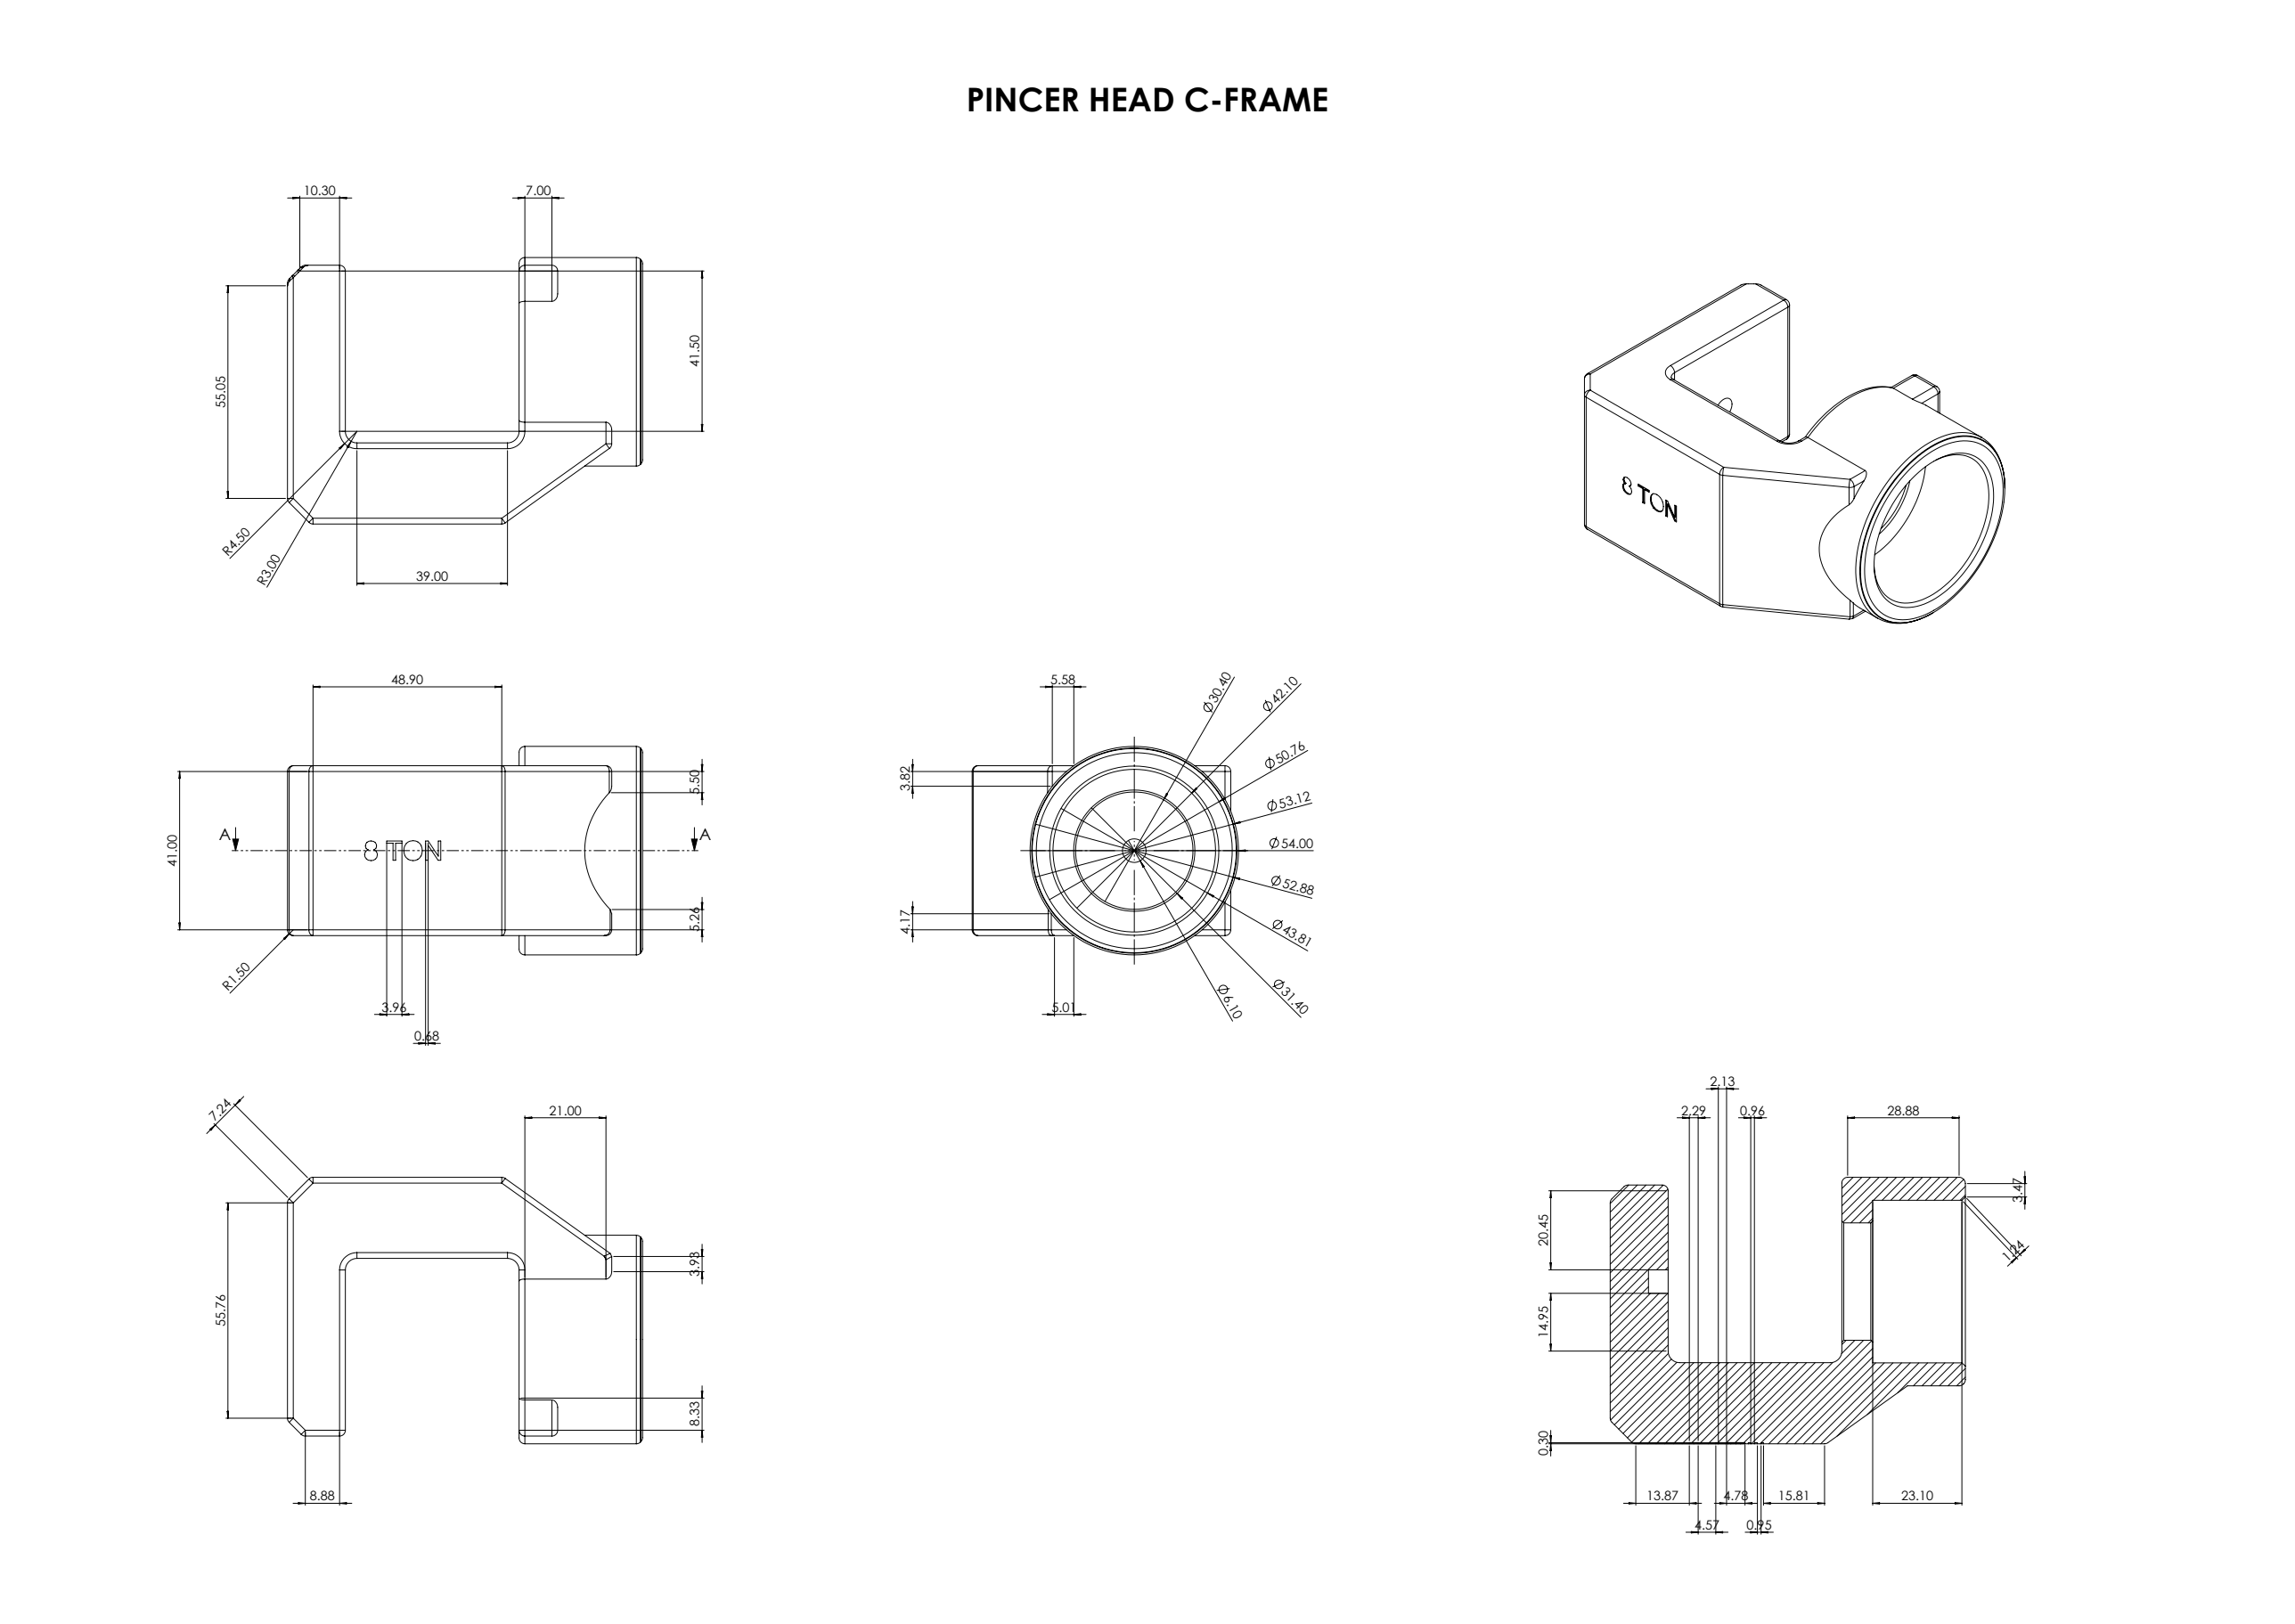
ISO-10303-21;
HEADER;
/* Generated by software containing ST-Developer
 * from STEP Tools, Inc. (www.steptools.com) 
 */

FILE_DESCRIPTION(
/* description */ (''),
/* implementation_level */ '2;1');

FILE_NAME(
/* name */ '01_Pincer_Head_C-Frame.step',
/* time_stamp */ '2026-10-26T03:55:20-07:00',
/* author */ (''),
/* organization */ (''),
/* preprocessor_version */ 'ST-DEVELOPER v20.2',
/* originating_system */ 'Autodesk Translation Framework v15.15.0.0',
/* authorisation */ '');

FILE_SCHEMA (('AUTOMOTIVE_DESIGN { 1 0 10303 214 3 1 1 }'));
ENDSEC;

DATA;
#10=MECHANICAL_DESIGN_GEOMETRIC_PRESENTATION_REPRESENTATION('',(#175),#45236);
#135=SHAPE_REPRESENTATION_RELATIONSHIP('SRR','None',#45314,#155);
#155=ADVANCED_BREP_SHAPE_REPRESENTATION('',(#195),#45216);
#175=STYLED_ITEM('',(#45463),#195);
#195=MANIFOLD_SOLID_BREP('Body1',#16517);
#215=TOROIDAL_SURFACE('',#16890,25.3786796564404,1.5);
#216=TOROIDAL_SURFACE('',#16900,25.5,1.5);
#217=TOROIDAL_SURFACE('',#16910,25.5,1.5);
#218=TOROIDAL_SURFACE('',#16914,4.5,1.5);
#219=TOROIDAL_SURFACE('',#16920,4.5,1.5);
#220=TOROIDAL_SURFACE('',#16924,4.5,1.5);
#221=TOROIDAL_SURFACE('',#16926,25.5,1.5);
#222=TOROIDAL_SURFACE('',#16927,4.5,1.5);
#223=TOROIDAL_SURFACE('',#16932,25.5,1.5);
#231=SPHERICAL_SURFACE('',#16793,1.5);
#232=SPHERICAL_SURFACE('',#16796,1.5);
#233=SPHERICAL_SURFACE('',#16802,1.5);
#234=SPHERICAL_SURFACE('',#16808,1.5);
#235=SPHERICAL_SURFACE('',#16812,1.5);
#236=SPHERICAL_SURFACE('',#16817,1.5);
#237=SPHERICAL_SURFACE('',#16821,1.5);
#238=SPHERICAL_SURFACE('',#16827,1.5);
#239=SPHERICAL_SURFACE('',#16830,1.5);
#240=SPHERICAL_SURFACE('',#16836,1.5);
#241=SPHERICAL_SURFACE('',#16842,1.5);
#242=SPHERICAL_SURFACE('',#16848,1.5);
#243=SPHERICAL_SURFACE('',#16853,1.5);
#244=SPHERICAL_SURFACE('',#16874,1.5);
#245=SPHERICAL_SURFACE('',#16880,1.5);
#246=ELLIPSE('',#16775,30.3654774451956,27.);
#247=ELLIPSE('',#16782,46.4525564420302,27.);
#256=B_SPLINE_CURVE_WITH_KNOTS('',3,(#22232,#22233,#22234,#22235,#22236,
#22237,#22238,#22239,#22240,#22241,#22242,#22243,#22244,#22245,#22246,#22247,
#22248,#22249,#22250,#22251,#22252,#22253,#22254,#22255,#22256,#22257,#22258,
#22259,#22260,#22261,#22262,#22263,#22264,#22265,#22266,#22267,#22268,#22269,
#22270,#22271,#22272,#22273,#22274,#22275,#22276,#22277,#22278,#22279,#22280,
#22281,#22282,#22283,#22284,#22285,#22286),.UNSPECIFIED.,.F.,.F.,(4,3,3,
3,3,3,3,3,3,3,3,3,3,3,3,3,3,3,4),(0.,0.045710607901934,0.0936977578945001,
0.144847111669027,0.20140314890997,0.272909847076527,0.34684212796304,0.403542711042019,
0.454759213428076,0.503663771096975,0.553082777660006,0.60625025134459,
0.667135318470237,0.750351488852678,0.812763616639508,0.865509180697515,
0.91510065731714,0.961342755203381,1.),.UNSPECIFIED.);
#257=B_SPLINE_CURVE_WITH_KNOTS('',3,(#22288,#22289,#22290,#22291),
 .UNSPECIFIED.,.F.,.F.,(4,4),(0.,1.),.UNSPECIFIED.);
#258=B_SPLINE_CURVE_WITH_KNOTS('',3,(#22293,#22294,#22295,#22296,#22297,
#22298,#22299,#22300,#22301,#22302,#22303,#22304,#22305,#22306,#22307,#22308,
#22309,#22310,#22311,#22312,#22313,#22314,#22315,#22316,#22317,#22318,#22319,
#22320,#22321,#22322,#22323,#22324,#22325,#22326,#22327,#22328,#22329,#22330,
#22331,#22332,#22333,#22334,#22335,#22336,#22337,#22338,#22339,#22340,#22341,
#22342,#22343,#22344,#22345,#22346,#22347),.UNSPECIFIED.,.F.,.F.,(4,3,3,
3,3,3,3,3,3,3,3,3,3,3,3,3,3,3,4),(0.,0.0457165824991635,0.0937104844515761,
0.144867913797289,0.201436011576242,0.27297908229306,0.346880659378771,
0.403581201094802,0.454799677982589,0.503723597905468,0.553141531246011,
0.606309913173532,0.667202763475632,0.750402072606724,0.812801554455043,
0.865537008236129,0.915120309500579,0.961355859688362,1.),.UNSPECIFIED.);
#259=B_SPLINE_CURVE_WITH_KNOTS('',3,(#22370,#22371,#22372,#22373,#22374),
 .UNSPECIFIED.,.F.,.F.,(4,1,4),(-1.66265780683826,-0.950090175336147,8.76618254786689E-34),
 .UNSPECIFIED.);
#260=B_SPLINE_CURVE_WITH_KNOTS('',3,(#22377,#22378,#22379,#22380,#22381),
 .UNSPECIFIED.,.F.,.F.,(4,1,4),(-8.76618254786689E-34,0.950090175336147,
1.66265780683826),.UNSPECIFIED.);
#261=B_SPLINE_CURVE_WITH_KNOTS('',3,(#22452,#22453,#22454,#22455,#22456,
#22457,#22458,#22459,#22460,#22461,#22462,#22463,#22464,#22465,#22466,#22467,
#22468,#22469,#22470,#22471,#22472,#22473,#22474,#22475,#22476,#22477,#22478,
#22479,#22480,#22481,#22482,#22483,#22484,#22485,#22486,#22487,#22488,#22489,
#22490,#22491,#22492,#22493,#22494,#22495,#22496,#22497,#22498,#22499,#22500,
#22501,#22502,#22503,#22504,#22505,#22506),.UNSPECIFIED.,.F.,.F.,(4,3,3,
3,3,3,3,3,3,3,3,3,3,3,3,3,3,3,4),(0.,0.0454739962515773,0.0931998981823239,
0.144047233375039,0.200179420009566,0.270609269371814,0.345305256937859,
0.401904934183246,0.452978957125852,0.503375918080837,0.552516920031195,
0.605334615481369,0.665679077650195,0.749259308237646,0.811944481178235,
0.864470546131162,0.91385478632005,0.959883517726927,1.),.UNSPECIFIED.);
#262=B_SPLINE_CURVE_WITH_KNOTS('',3,(#22508,#22509,#22510,#22511),
 .UNSPECIFIED.,.F.,.F.,(4,4),(-1.,0.),.UNSPECIFIED.);
#263=B_SPLINE_CURVE_WITH_KNOTS('',3,(#22513,#22514,#22515,#22516,#22517,
#22518,#22519,#22520,#22521,#22522,#22523,#22524,#22525,#22526,#22527,#22528,
#22529,#22530,#22531,#22532,#22533,#22534,#22535,#22536,#22537,#22538,#22539,
#22540,#22541,#22542,#22543,#22544,#22545,#22546,#22547,#22548,#22549,#22550,
#22551,#22552,#22553,#22554,#22555,#22556,#22557,#22558,#22559,#22560,#22561,
#22562,#22563,#22564,#22565,#22566,#22567),.UNSPECIFIED.,.F.,.F.,(4,3,3,
3,3,3,3,3,3,3,3,3,3,3,3,3,3,3,4),(0.,0.0454759500687694,0.0932040608878028,
0.144054037760376,0.200190152021456,0.270631477875933,0.345316813881959,
0.401916574351127,0.452991295574466,0.503400827180246,0.552541816304096,
0.605360167195349,0.665708324703348,0.749281243527511,0.811960932645634,
0.864483394812729,0.913864760430574,0.959891262991555,1.),.UNSPECIFIED.);
#264=B_SPLINE_CURVE_WITH_KNOTS('',3,(#22595,#22596,#22597,#22598,#22599,
#22600,#22601,#22602,#22603,#22604,#22605,#22606,#22607,#22608,#22609,#22610,
#22611,#22612,#22613,#22614,#22615,#22616,#22617,#22618,#22619,#22620,#22621,
#22622,#22623,#22624,#22625,#22626,#22627,#22628,#22629,#22630,#22631,#22632,
#22633,#22634,#22635,#22636,#22637,#22638,#22639,#22640,#22641,#22642,#22643,
#22644,#22645,#22646,#22647,#22648,#22649),.UNSPECIFIED.,.F.,.F.,(4,3,3,
3,3,3,3,3,3,3,3,3,3,3,3,3,3,3,4),(0.,0.0454739962517236,0.0931998981821424,
0.144047233377289,0.200179420014148,0.270609269376805,0.345305256939856,
0.401904934184723,0.452978957126951,0.503375918082738,0.552516920034218,
0.605334615484988,0.665679077654914,0.749259308241186,0.811944481180889,
0.864470546134333,0.913854786323009,0.959883517729389,1.),.UNSPECIFIED.);
#265=B_SPLINE_CURVE_WITH_KNOTS('',3,(#22651,#22652,#22653,#22654),
 .UNSPECIFIED.,.F.,.F.,(4,4),(0.,1.),.UNSPECIFIED.);
#266=B_SPLINE_CURVE_WITH_KNOTS('',3,(#22656,#22657,#22658,#22659,#22660,
#22661,#22662,#22663,#22664,#22665,#22666,#22667,#22668,#22669,#22670,#22671,
#22672,#22673,#22674,#22675,#22676,#22677,#22678,#22679,#22680,#22681,#22682,
#22683,#22684,#22685,#22686,#22687,#22688,#22689,#22690,#22691,#22692,#22693,
#22694,#22695,#22696,#22697,#22698,#22699,#22700,#22701,#22702,#22703,#22704,
#22705,#22706,#22707,#22708,#22709,#22710),.UNSPECIFIED.,.F.,.F.,(4,3,3,
3,3,3,3,3,3,3,3,3,3,3,3,3,3,3,4),(0.,0.0454759500669044,0.0932040608838389,
0.144054037755869,0.200190152008621,0.270631477848411,0.345316813870146,
0.401916574343999,0.4529912955674,0.503400827166756,0.552541816289859,0.605360167180691,
0.665708324686459,0.749281243514844,0.811960932636133,0.864483394804765,
0.913864760422638,0.959891262983851,1.),.UNSPECIFIED.);
#267=B_SPLINE_CURVE_WITH_KNOTS('',3,(#22729,#22730,#22731,#22732),
 .UNSPECIFIED.,.F.,.F.,(4,4),(1.38548660592135,2.14032342811115),
 .UNSPECIFIED.);
#268=B_SPLINE_CURVE_WITH_KNOTS('',3,(#22735,#22736,#22737,#22738),
 .UNSPECIFIED.,.F.,.F.,(4,4),(-2.14032342811115,-1.38548660592135),
 .UNSPECIFIED.);
#269=B_SPLINE_CURVE_WITH_KNOTS('',3,(#22759,#22760,#22761,#22762),
 .UNSPECIFIED.,.F.,.F.,(4,4),(-1.33701776267244,-0.785398163397445),
 .UNSPECIFIED.);
#270=B_SPLINE_CURVE_WITH_KNOTS('',3,(#22765,#22766,#22767,#22768),
 .UNSPECIFIED.,.F.,.F.,(4,4),(0.785398163397445,1.33701776267244),
 .UNSPECIFIED.);
#271=B_SPLINE_CURVE_WITH_KNOTS('',3,(#22785,#22786,#22787,#22788),
 .UNSPECIFIED.,.F.,.F.,(4,4),(-2.35619449019235,-2.14032342811107),
 .UNSPECIFIED.);
#272=B_SPLINE_CURVE_WITH_KNOTS('',3,(#22789,#22790,#22791,#22792),
 .UNSPECIFIED.,.F.,.F.,(4,4),(2.14032342811107,2.35619449019235),
 .UNSPECIFIED.);
#273=B_SPLINE_CURVE_WITH_KNOTS('',3,(#22818,#22819,#22820,#22821),
 .UNSPECIFIED.,.F.,.F.,(4,4),(-1.5707963267949,-1.33701776267243),
 .UNSPECIFIED.);
#274=B_SPLINE_CURVE_WITH_KNOTS('',3,(#22822,#22823,#22824,#22825),
 .UNSPECIFIED.,.F.,.F.,(4,4),(1.33701776267243,1.5707963267949),
 .UNSPECIFIED.);
#275=B_SPLINE_CURVE_WITH_KNOTS('',3,(#22846,#22847,#22848,#22849),
 .UNSPECIFIED.,.F.,.F.,(4,4),(-1.33701776267244,-0.785398163397449),
 .UNSPECIFIED.);
#276=B_SPLINE_CURVE_WITH_KNOTS('',3,(#22852,#22853,#22854,#22855),
 .UNSPECIFIED.,.F.,.F.,(4,4),(0.785398163397449,1.33701776267244),
 .UNSPECIFIED.);
#277=B_SPLINE_CURVE_WITH_KNOTS('',3,(#22872,#22873,#22874,#22875),
 .UNSPECIFIED.,.F.,.F.,(4,4),(1.33701776267244,1.5707963267949),
 .UNSPECIFIED.);
#278=B_SPLINE_CURVE_WITH_KNOTS('',3,(#22876,#22877,#22878,#22879),
 .UNSPECIFIED.,.F.,.F.,(4,4),(-1.5707963267949,-1.33701776267244),
 .UNSPECIFIED.);
#279=B_SPLINE_CURVE_WITH_KNOTS('',3,(#22897,#22898,#22899,#22900),
 .UNSPECIFIED.,.F.,.F.,(4,4),(1.38548660592135,2.14032342811115),
 .UNSPECIFIED.);
#280=B_SPLINE_CURVE_WITH_KNOTS('',3,(#22903,#22904,#22905,#22906),
 .UNSPECIFIED.,.F.,.F.,(4,4),(-2.14032342811115,-1.38548660592135),
 .UNSPECIFIED.);
#281=B_SPLINE_CURVE_WITH_KNOTS('',3,(#22923,#22924,#22925,#22926),
 .UNSPECIFIED.,.F.,.F.,(4,4),(2.14032342811108,2.35619449019234),
 .UNSPECIFIED.);
#282=B_SPLINE_CURVE_WITH_KNOTS('',3,(#22927,#22928,#22929,#22930),
 .UNSPECIFIED.,.F.,.F.,(4,4),(-2.35619449019234,-2.14032342811108),
 .UNSPECIFIED.);
#283=B_SPLINE_CURVE_WITH_KNOTS('',3,(#22971,#22972,#22973,#22974,#22975,
#22976,#22977,#22978,#22979,#22980,#22981,#22982),.UNSPECIFIED.,.F.,.F.,
(4,2,2,2,2,4),(0.,0.0283853554165653,0.0567707108331306,0.113541421666261,
0.206773466476135,0.300005511286008),.UNSPECIFIED.);
#284=B_SPLINE_CURVE_WITH_KNOTS('',3,(#22988,#22989,#22990,#22991,#22992,
#22993,#22994,#22995,#22996,#22997),.UNSPECIFIED.,.F.,.F.,(4,2,2,2,4),(0.328734721229726,
0.593926356430402,0.667111024695369,0.687829707063932,0.708548389432494),
 .UNSPECIFIED.);
#285=B_SPLINE_CURVE_WITH_KNOTS('',3,(#23011,#23012,#23013,#23014,#23015,
#23016,#23017,#23018),.UNSPECIFIED.,.F.,.F.,(4,2,2,4),(0.894852523096926,
0.994118550241906,1.09338457738688,1.10550146254272),.UNSPECIFIED.);
#286=B_SPLINE_CURVE_WITH_KNOTS('',3,(#23023,#23024,#23025,#23026,#23027,
#23028,#23029,#23030,#23031,#23032,#23033,#23034),.UNSPECIFIED.,.F.,.F.,
(4,2,2,2,2,4),(0.,0.0283853554165652,0.0567707108331305,0.113541421666261,
0.206773466476134,0.300005511286007),.UNSPECIFIED.);
#287=B_SPLINE_CURVE_WITH_KNOTS('',2,(#23117,#23118,#23119),
 .UNSPECIFIED.,.F.,.F.,(3,3),(0.,1.),.UNSPECIFIED.);
#288=B_SPLINE_CURVE_WITH_KNOTS('',2,(#23121,#23122,#23123),
 .UNSPECIFIED.,.F.,.F.,(3,3),(0.,1.),.UNSPECIFIED.);
#289=B_SPLINE_CURVE_WITH_KNOTS('',2,(#23125,#23126,#23127),
 .UNSPECIFIED.,.F.,.F.,(3,3),(0.,1.),.UNSPECIFIED.);
#290=B_SPLINE_CURVE_WITH_KNOTS('',2,(#23129,#23130,#23131),
 .UNSPECIFIED.,.F.,.F.,(3,3),(0.,1.),.UNSPECIFIED.);
#291=B_SPLINE_CURVE_WITH_KNOTS('',2,(#23133,#23134,#23135),
 .UNSPECIFIED.,.F.,.F.,(3,3),(0.,1.),.UNSPECIFIED.);
#292=B_SPLINE_CURVE_WITH_KNOTS('',2,(#23137,#23138,#23139),
 .UNSPECIFIED.,.F.,.F.,(3,3),(0.,1.),.UNSPECIFIED.);
#293=B_SPLINE_CURVE_WITH_KNOTS('',2,(#23141,#23142,#23143),
 .UNSPECIFIED.,.F.,.F.,(3,3),(0.,1.),.UNSPECIFIED.);
#294=B_SPLINE_CURVE_WITH_KNOTS('',2,(#23145,#23146,#23147),
 .UNSPECIFIED.,.F.,.F.,(3,3),(0.,1.),.UNSPECIFIED.);
#295=B_SPLINE_CURVE_WITH_KNOTS('',2,(#23149,#23150,#23151),
 .UNSPECIFIED.,.F.,.F.,(3,3),(0.,1.),.UNSPECIFIED.);
#296=B_SPLINE_CURVE_WITH_KNOTS('',2,(#23153,#23154,#23155),
 .UNSPECIFIED.,.F.,.F.,(3,3),(0.,1.),.UNSPECIFIED.);
#297=B_SPLINE_CURVE_WITH_KNOTS('',2,(#23156,#23157,#23158),
 .UNSPECIFIED.,.F.,.F.,(3,3),(0.,1.),.UNSPECIFIED.);
#298=B_SPLINE_CURVE_WITH_KNOTS('',2,(#23177,#23178,#23179),
 .UNSPECIFIED.,.F.,.F.,(3,3),(0.,1.),.UNSPECIFIED.);
#299=B_SPLINE_CURVE_WITH_KNOTS('',2,(#23181,#23182,#23183),
 .UNSPECIFIED.,.F.,.F.,(3,3),(0.,1.),.UNSPECIFIED.);
#300=B_SPLINE_CURVE_WITH_KNOTS('',2,(#23185,#23186,#23187),
 .UNSPECIFIED.,.F.,.F.,(3,3),(0.,1.),.UNSPECIFIED.);
#301=B_SPLINE_CURVE_WITH_KNOTS('',2,(#23189,#23190,#23191),
 .UNSPECIFIED.,.F.,.F.,(3,3),(0.,1.),.UNSPECIFIED.);
#302=B_SPLINE_CURVE_WITH_KNOTS('',2,(#23193,#23194,#23195),
 .UNSPECIFIED.,.F.,.F.,(3,3),(0.,1.),.UNSPECIFIED.);
#303=B_SPLINE_CURVE_WITH_KNOTS('',2,(#23197,#23198,#23199),
 .UNSPECIFIED.,.F.,.F.,(3,3),(0.,1.),.UNSPECIFIED.);
#304=B_SPLINE_CURVE_WITH_KNOTS('',2,(#23201,#23202,#23203),
 .UNSPECIFIED.,.F.,.F.,(3,3),(0.,1.),.UNSPECIFIED.);
#305=B_SPLINE_CURVE_WITH_KNOTS('',2,(#23205,#23206,#23207),
 .UNSPECIFIED.,.F.,.F.,(3,3),(0.,1.),.UNSPECIFIED.);
#306=B_SPLINE_CURVE_WITH_KNOTS('',2,(#23209,#23210,#23211),
 .UNSPECIFIED.,.F.,.F.,(3,3),(0.,1.),.UNSPECIFIED.);
#307=B_SPLINE_CURVE_WITH_KNOTS('',2,(#23213,#23214,#23215),
 .UNSPECIFIED.,.F.,.F.,(3,3),(0.,1.),.UNSPECIFIED.);
#308=B_SPLINE_CURVE_WITH_KNOTS('',2,(#23217,#23218,#23219),
 .UNSPECIFIED.,.F.,.F.,(3,3),(0.,1.),.UNSPECIFIED.);
#309=B_SPLINE_CURVE_WITH_KNOTS('',2,(#23221,#23222,#23223),
 .UNSPECIFIED.,.F.,.F.,(3,3),(0.,1.),.UNSPECIFIED.);
#310=B_SPLINE_CURVE_WITH_KNOTS('',2,(#23225,#23226,#23227),
 .UNSPECIFIED.,.F.,.F.,(3,3),(0.,1.),.UNSPECIFIED.);
#311=B_SPLINE_CURVE_WITH_KNOTS('',2,(#23229,#23230,#23231),
 .UNSPECIFIED.,.F.,.F.,(3,3),(0.,1.),.UNSPECIFIED.);
#312=B_SPLINE_CURVE_WITH_KNOTS('',2,(#23233,#23234,#23235),
 .UNSPECIFIED.,.F.,.F.,(3,3),(0.,1.),.UNSPECIFIED.);
#313=B_SPLINE_CURVE_WITH_KNOTS('',2,(#23236,#23237,#23238),
 .UNSPECIFIED.,.F.,.F.,(3,3),(0.,1.),.UNSPECIFIED.);
#314=B_SPLINE_CURVE_WITH_KNOTS('',3,(#23280,#23281,#23282,#23283,#23284,
#23285,#23286,#23287,#23288,#23289,#23290,#23291),.UNSPECIFIED.,.F.,.F.,
(4,2,2,2,2,4),(-0.300005511286007,-0.206773466476134,-0.113541421666261,
-0.0567707108331306,-0.0283853554165654,0.),.UNSPECIFIED.);
#315=B_SPLINE_CURVE_WITH_KNOTS('',3,(#23300,#23301,#23302,#23303,#23304,
#23305,#23306,#23307,#23308,#23309,#23310,#23311,#23312,#23313),
 .UNSPECIFIED.,.F.,.F.,(4,2,2,2,2,2,4),(-0.242126305586689,-0.241475938992465,
-0.207325141862153,-0.17328250313445,-0.113202201999937,-0.0559588482258517,
0.),.UNSPECIFIED.);
#316=B_SPLINE_CURVE_WITH_KNOTS('',3,(#23315,#23316,#23317,#23318,#23319,
#23320,#23321,#23322,#23323,#23324,#23325,#23326,#23327,#23328),
 .UNSPECIFIED.,.F.,.F.,(4,2,2,2,2,2,4),(-0.237971793841113,-0.180365854109777,
-0.122215701674832,-0.0629296381239613,-0.0314884565302302,0.,0.000668991455295416),
 .UNSPECIFIED.);
#317=B_SPLINE_CURVE_WITH_KNOTS('',3,(#23339,#23340,#23341,#23342,#23343,
#23344,#23345,#23346,#23347,#23348,#23349,#23350,#23351,#23352),
 .UNSPECIFIED.,.F.,.F.,(4,2,2,2,2,2,4),(-0.23846990825455,-0.237798685175548,
-0.20633335283318,-0.174914932942728,-0.115672316276476,-0.0575645322663487,
0.),.UNSPECIFIED.);
#318=B_SPLINE_CURVE_WITH_KNOTS('',3,(#23356,#23357,#23358,#23359,#23360,
#23361,#23362,#23363,#23364,#23365,#23366,#23367,#23368,#23369),
 .UNSPECIFIED.,.F.,.F.,(4,2,2,2,2,2,4),(-0.241896356494029,-0.185842740394847,
-0.128518974500819,-0.0683631385924297,-0.0342301099048936,0.,0.000659700792702867),
 .UNSPECIFIED.);
#319=B_SPLINE_CURVE_WITH_KNOTS('',3,(#23388,#23389,#23390,#23391,#23392,
#23393,#23394,#23395,#23396,#23397),.UNSPECIFIED.,.F.,.F.,(4,2,2,2,4),(0.712943458944601,
0.733662141313163,0.754380823681726,0.827565491946693,1.09275712714737),
 .UNSPECIFIED.);
#320=B_SPLINE_CURVE_WITH_KNOTS('',3,(#23402,#23403,#23404,#23405,#23406,
#23407,#23408,#23409,#23410,#23411,#23412,#23413),.UNSPECIFIED.,.F.,.F.,
(4,2,2,2,2,4),(-0.300005511286008,-0.206773466476135,-0.113541421666261,
-0.0567707108331308,-0.0283853554165654,0.),.UNSPECIFIED.);
#321=B_SPLINE_CURVE_WITH_KNOTS('',3,(#23474,#23475,#23476,#23477,#23478,
#23479,#23480,#23481,#23482,#23483,#23484,#23485,#23486,#23487),
 .UNSPECIFIED.,.F.,.F.,(4,2,2,2,2,2,4),(-0.000578412997427686,0.,0.0341328715078763,
0.0680999028359124,0.128446519154858,0.185899361060066,0.241981137339067),
 .UNSPECIFIED.);
#322=B_SPLINE_CURVE_WITH_KNOTS('',3,(#23498,#23499,#23500,#23501,#23502,
#23503,#23504,#23505,#23506,#23507,#23508,#23509,#23510,#23511),
 .UNSPECIFIED.,.F.,.F.,(4,2,2,2,2,2,4),(0.,0.0559818727072018,0.113332368636633,
0.173571484036089,0.207478006800184,0.241550074317809,0.242127456935271),
 .UNSPECIFIED.);
#323=B_SPLINE_CURVE_WITH_KNOTS('',2,(#23531,#23532,#23533),
 .UNSPECIFIED.,.F.,.F.,(3,3),(0.,1.),.UNSPECIFIED.);
#324=B_SPLINE_CURVE_WITH_KNOTS('',2,(#23543,#23544,#23545),
 .UNSPECIFIED.,.F.,.F.,(3,3),(0.,1.),.UNSPECIFIED.);
#325=B_SPLINE_CURVE_WITH_KNOTS('',2,(#23554,#23555,#23556),
 .UNSPECIFIED.,.F.,.F.,(3,3),(0.,1.),.UNSPECIFIED.);
#326=B_SPLINE_CURVE_WITH_KNOTS('',2,(#23565,#23566,#23567),
 .UNSPECIFIED.,.F.,.F.,(3,3),(0.,1.),.UNSPECIFIED.);
#327=B_SPLINE_CURVE_WITH_KNOTS('',2,(#23576,#23577,#23578),
 .UNSPECIFIED.,.F.,.F.,(3,3),(0.,1.),.UNSPECIFIED.);
#328=B_SPLINE_CURVE_WITH_KNOTS('',2,(#23587,#23588,#23589),
 .UNSPECIFIED.,.F.,.F.,(3,3),(0.,1.),.UNSPECIFIED.);
#329=B_SPLINE_CURVE_WITH_KNOTS('',2,(#23598,#23599,#23600),
 .UNSPECIFIED.,.F.,.F.,(3,3),(0.,1.),.UNSPECIFIED.);
#330=B_SPLINE_CURVE_WITH_KNOTS('',2,(#23609,#23610,#23611),
 .UNSPECIFIED.,.F.,.F.,(3,3),(0.,1.),.UNSPECIFIED.);
#331=B_SPLINE_CURVE_WITH_KNOTS('',2,(#23620,#23621,#23622),
 .UNSPECIFIED.,.F.,.F.,(3,3),(0.,1.),.UNSPECIFIED.);
#332=B_SPLINE_CURVE_WITH_KNOTS('',2,(#23631,#23632,#23633),
 .UNSPECIFIED.,.F.,.F.,(3,3),(0.,1.),.UNSPECIFIED.);
#333=B_SPLINE_CURVE_WITH_KNOTS('',2,(#23640,#23641,#23642),
 .UNSPECIFIED.,.F.,.F.,(3,3),(0.,1.),.UNSPECIFIED.);
#334=B_SPLINE_CURVE_WITH_KNOTS('',2,(#23686,#23687,#23688),
 .UNSPECIFIED.,.F.,.F.,(3,3),(0.,1.),.UNSPECIFIED.);
#335=B_SPLINE_CURVE_WITH_KNOTS('',2,(#23698,#23699,#23700),
 .UNSPECIFIED.,.F.,.F.,(3,3),(0.,1.),.UNSPECIFIED.);
#336=B_SPLINE_CURVE_WITH_KNOTS('',2,(#23709,#23710,#23711),
 .UNSPECIFIED.,.F.,.F.,(3,3),(0.,1.),.UNSPECIFIED.);
#337=B_SPLINE_CURVE_WITH_KNOTS('',2,(#23720,#23721,#23722),
 .UNSPECIFIED.,.F.,.F.,(3,3),(0.,1.),.UNSPECIFIED.);
#338=B_SPLINE_CURVE_WITH_KNOTS('',2,(#23731,#23732,#23733),
 .UNSPECIFIED.,.F.,.F.,(3,3),(0.,1.),.UNSPECIFIED.);
#339=B_SPLINE_CURVE_WITH_KNOTS('',2,(#23742,#23743,#23744),
 .UNSPECIFIED.,.F.,.F.,(3,3),(0.,1.),.UNSPECIFIED.);
#340=B_SPLINE_CURVE_WITH_KNOTS('',2,(#23753,#23754,#23755),
 .UNSPECIFIED.,.F.,.F.,(3,3),(0.,1.),.UNSPECIFIED.);
#341=B_SPLINE_CURVE_WITH_KNOTS('',2,(#23764,#23765,#23766),
 .UNSPECIFIED.,.F.,.F.,(3,3),(0.,1.),.UNSPECIFIED.);
#342=B_SPLINE_CURVE_WITH_KNOTS('',2,(#23775,#23776,#23777),
 .UNSPECIFIED.,.F.,.F.,(3,3),(0.,1.),.UNSPECIFIED.);
#343=B_SPLINE_CURVE_WITH_KNOTS('',2,(#23786,#23787,#23788),
 .UNSPECIFIED.,.F.,.F.,(3,3),(0.,1.),.UNSPECIFIED.);
#344=B_SPLINE_CURVE_WITH_KNOTS('',2,(#23797,#23798,#23799),
 .UNSPECIFIED.,.F.,.F.,(3,3),(0.,1.),.UNSPECIFIED.);
#345=B_SPLINE_CURVE_WITH_KNOTS('',2,(#23808,#23809,#23810),
 .UNSPECIFIED.,.F.,.F.,(3,3),(0.,1.),.UNSPECIFIED.);
#346=B_SPLINE_CURVE_WITH_KNOTS('',2,(#23819,#23820,#23821),
 .UNSPECIFIED.,.F.,.F.,(3,3),(0.,1.),.UNSPECIFIED.);
#347=B_SPLINE_CURVE_WITH_KNOTS('',2,(#23830,#23831,#23832),
 .UNSPECIFIED.,.F.,.F.,(3,3),(0.,1.),.UNSPECIFIED.);
#348=B_SPLINE_CURVE_WITH_KNOTS('',2,(#23841,#23842,#23843),
 .UNSPECIFIED.,.F.,.F.,(3,3),(0.,1.),.UNSPECIFIED.);
#349=B_SPLINE_CURVE_WITH_KNOTS('',2,(#23850,#23851,#23852),
 .UNSPECIFIED.,.F.,.F.,(3,3),(0.,1.),.UNSPECIFIED.);
#814=B_SPLINE_SURFACE_WITH_KNOTS('',3,3,((#22206,#22207,#22208,#22209,#22210,
#22211),(#22212,#22213,#22214,#22215,#22216,#22217),(#22218,#22219,#22220,
#22221,#22222,#22223),(#22224,#22225,#22226,#22227,#22228,#22229)),
 .UNSPECIFIED.,.F.,.F.,.F.,(4,4),(4,1,1,4),(0.,1.),(0.,0.571428571428571,
0.857142857142857,1.),.UNSPECIFIED.);
#815=B_SPLINE_SURFACE_WITH_KNOTS('',3,3,((#22349,#22350,#22351,#22352,#22353),
(#22354,#22355,#22356,#22357,#22358),(#22359,#22360,#22361,#22362,#22363),
(#22364,#22365,#22366,#22367,#22368)),.UNSPECIFIED.,.F.,.F.,.F.,(4,4),(4,
1,4),(0.,1.),(-1.66265780683826,-0.950090175336147,8.76618254786689E-34),
 .UNSPECIFIED.);
#816=B_SPLINE_SURFACE_WITH_KNOTS('',3,3,((#22426,#22427,#22428,#22429,#22430,
#22431),(#22432,#22433,#22434,#22435,#22436,#22437),(#22438,#22439,#22440,
#22441,#22442,#22443),(#22444,#22445,#22446,#22447,#22448,#22449)),
 .UNSPECIFIED.,.F.,.F.,.F.,(4,4),(4,1,1,4),(0.,1.),(0.,0.571428571428571,
0.857142857142857,1.),.UNSPECIFIED.);
#817=B_SPLINE_SURFACE_WITH_KNOTS('',3,3,((#22569,#22570,#22571,#22572,#22573,
#22574),(#22575,#22576,#22577,#22578,#22579,#22580),(#22581,#22582,#22583,
#22584,#22585,#22586),(#22587,#22588,#22589,#22590,#22591,#22592)),
 .UNSPECIFIED.,.F.,.F.,.F.,(4,4),(4,1,1,4),(0.,1.),(0.,0.571428571428571,
0.857142857142857,1.),.UNSPECIFIED.);
#818=B_SPLINE_SURFACE_WITH_KNOTS('',3,3,((#22712,#22713,#22714,#22715),
(#22716,#22717,#22718,#22719),(#22720,#22721,#22722,#22723),(#22724,#22725,
#22726,#22727)),.UNSPECIFIED.,.F.,.F.,.F.,(4,4),(4,4),(0.,1.),(1.38548660592135,
2.14032342811115),.UNSPECIFIED.);
#819=B_SPLINE_SURFACE_WITH_KNOTS('',3,3,((#22739,#22740,#22741,#22742),
(#22743,#22744,#22745,#22746),(#22747,#22748,#22749,#22750),(#22751,#22752,
#22753,#22754)),.UNSPECIFIED.,.F.,.F.,.F.,(4,4),(4,4),(0.,1.),(-1.33701776267244,
-0.785398163397445),.UNSPECIFIED.);
#820=B_SPLINE_SURFACE_WITH_KNOTS('',3,3,((#22769,#22770,#22771,#22772),
(#22773,#22774,#22775,#22776),(#22777,#22778,#22779,#22780),(#22781,#22782,
#22783,#22784)),.UNSPECIFIED.,.F.,.F.,.F.,(4,4),(4,4),(0.,1.),(2.14032342811107,
2.35619449019235),.UNSPECIFIED.);
#821=B_SPLINE_SURFACE_WITH_KNOTS('',3,3,((#22802,#22803,#22804,#22805),
(#22806,#22807,#22808,#22809),(#22810,#22811,#22812,#22813),(#22814,#22815,
#22816,#22817)),.UNSPECIFIED.,.F.,.F.,.F.,(4,4),(4,4),(0.,1.),(1.33701776267243,
1.5707963267949),.UNSPECIFIED.);
#822=B_SPLINE_SURFACE_WITH_KNOTS('',3,3,((#22826,#22827,#22828,#22829),
(#22830,#22831,#22832,#22833),(#22834,#22835,#22836,#22837),(#22838,#22839,
#22840,#22841)),.UNSPECIFIED.,.F.,.F.,.F.,(4,4),(4,4),(0.,1.),(0.785398163397449,
1.33701776267244),.UNSPECIFIED.);
#823=B_SPLINE_SURFACE_WITH_KNOTS('',3,3,((#22856,#22857,#22858,#22859),
(#22860,#22861,#22862,#22863),(#22864,#22865,#22866,#22867),(#22868,#22869,
#22870,#22871)),.UNSPECIFIED.,.F.,.F.,.F.,(4,4),(4,4),(0.,1.),(-1.5707963267949,
-1.33701776267244),.UNSPECIFIED.);
#824=B_SPLINE_SURFACE_WITH_KNOTS('',3,3,((#22880,#22881,#22882,#22883),
(#22884,#22885,#22886,#22887),(#22888,#22889,#22890,#22891),(#22892,#22893,
#22894,#22895)),.UNSPECIFIED.,.F.,.F.,.F.,(4,4),(4,4),(0.,1.),(-2.14032342811115,
-1.38548660592135),.UNSPECIFIED.);
#825=B_SPLINE_SURFACE_WITH_KNOTS('',3,3,((#22907,#22908,#22909,#22910),
(#22911,#22912,#22913,#22914),(#22915,#22916,#22917,#22918),(#22919,#22920,
#22921,#22922)),.UNSPECIFIED.,.F.,.F.,.F.,(4,4),(4,4),(0.,1.),(-2.35619449019234,
-2.14032342811108),.UNSPECIFIED.);
#826=B_SPLINE_SURFACE_WITH_KNOTS('',2,1,((#23522,#23523),(#23524,#23525),
(#23526,#23527)),.UNSPECIFIED.,.F.,.F.,.F.,(3,3),(2,2),(0.,1.),(0.,0.0300000000000002),
 .UNSPECIFIED.);
#827=B_SPLINE_SURFACE_WITH_KNOTS('',2,1,((#23535,#23536),(#23537,#23538),
(#23539,#23540)),.UNSPECIFIED.,.F.,.F.,.F.,(3,3),(2,2),(0.,1.),(0.,0.0300000000000002),
 .UNSPECIFIED.);
#828=B_SPLINE_SURFACE_WITH_KNOTS('',2,1,((#23546,#23547),(#23548,#23549),
(#23550,#23551)),.UNSPECIFIED.,.F.,.F.,.F.,(3,3),(2,2),(0.,1.),(0.,0.0300000000000002),
 .UNSPECIFIED.);
#829=B_SPLINE_SURFACE_WITH_KNOTS('',2,1,((#23557,#23558),(#23559,#23560),
(#23561,#23562)),.UNSPECIFIED.,.F.,.F.,.F.,(3,3),(2,2),(0.,1.),(0.,0.0300000000000002),
 .UNSPECIFIED.);
#830=B_SPLINE_SURFACE_WITH_KNOTS('',2,1,((#23568,#23569),(#23570,#23571),
(#23572,#23573)),.UNSPECIFIED.,.F.,.F.,.F.,(3,3),(2,2),(0.,1.),(0.,0.0300000000000002),
 .UNSPECIFIED.);
#831=B_SPLINE_SURFACE_WITH_KNOTS('',2,1,((#23579,#23580),(#23581,#23582),
(#23583,#23584)),.UNSPECIFIED.,.F.,.F.,.F.,(3,3),(2,2),(0.,1.),(0.,0.0300000000000002),
 .UNSPECIFIED.);
#832=B_SPLINE_SURFACE_WITH_KNOTS('',2,1,((#23590,#23591),(#23592,#23593),
(#23594,#23595)),.UNSPECIFIED.,.F.,.F.,.F.,(3,3),(2,2),(0.,1.),(0.,0.0300000000000002),
 .UNSPECIFIED.);
#833=B_SPLINE_SURFACE_WITH_KNOTS('',2,1,((#23601,#23602),(#23603,#23604),
(#23605,#23606)),.UNSPECIFIED.,.F.,.F.,.F.,(3,3),(2,2),(0.,1.),(0.,0.0300000000000002),
 .UNSPECIFIED.);
#834=B_SPLINE_SURFACE_WITH_KNOTS('',2,1,((#23612,#23613),(#23614,#23615),
(#23616,#23617)),.UNSPECIFIED.,.F.,.F.,.F.,(3,3),(2,2),(0.,1.),(0.,0.0300000000000002),
 .UNSPECIFIED.);
#835=B_SPLINE_SURFACE_WITH_KNOTS('',2,1,((#23623,#23624),(#23625,#23626),
(#23627,#23628)),.UNSPECIFIED.,.F.,.F.,.F.,(3,3),(2,2),(0.,1.),(0.,0.0300000000000002),
 .UNSPECIFIED.);
#836=B_SPLINE_SURFACE_WITH_KNOTS('',2,1,((#23634,#23635),(#23636,#23637),
(#23638,#23639)),.UNSPECIFIED.,.F.,.F.,.F.,(3,3),(2,2),(0.,1.),(0.,0.0300000000000002),
 .UNSPECIFIED.);
#837=B_SPLINE_SURFACE_WITH_KNOTS('',2,1,((#23677,#23678),(#23679,#23680),
(#23681,#23682)),.UNSPECIFIED.,.F.,.F.,.F.,(3,3),(2,2),(0.,1.),(0.,0.0300000000000002),
 .UNSPECIFIED.);
#838=B_SPLINE_SURFACE_WITH_KNOTS('',2,1,((#23690,#23691),(#23692,#23693),
(#23694,#23695)),.UNSPECIFIED.,.F.,.F.,.F.,(3,3),(2,2),(0.,1.),(0.,0.0300000000000002),
 .UNSPECIFIED.);
#839=B_SPLINE_SURFACE_WITH_KNOTS('',2,1,((#23701,#23702),(#23703,#23704),
(#23705,#23706)),.UNSPECIFIED.,.F.,.F.,.F.,(3,3),(2,2),(0.,1.),(0.,0.0300000000000002),
 .UNSPECIFIED.);
#840=B_SPLINE_SURFACE_WITH_KNOTS('',2,1,((#23712,#23713),(#23714,#23715),
(#23716,#23717)),.UNSPECIFIED.,.F.,.F.,.F.,(3,3),(2,2),(0.,1.),(0.,0.0300000000000002),
 .UNSPECIFIED.);
#841=B_SPLINE_SURFACE_WITH_KNOTS('',2,1,((#23723,#23724),(#23725,#23726),
(#23727,#23728)),.UNSPECIFIED.,.F.,.F.,.F.,(3,3),(2,2),(0.,1.),(0.,0.0300000000000002),
 .UNSPECIFIED.);
#842=B_SPLINE_SURFACE_WITH_KNOTS('',2,1,((#23734,#23735),(#23736,#23737),
(#23738,#23739)),.UNSPECIFIED.,.F.,.F.,.F.,(3,3),(2,2),(0.,1.),(0.,0.0300000000000002),
 .UNSPECIFIED.);
#843=B_SPLINE_SURFACE_WITH_KNOTS('',2,1,((#23745,#23746),(#23747,#23748),
(#23749,#23750)),.UNSPECIFIED.,.F.,.F.,.F.,(3,3),(2,2),(0.,1.),(0.,0.0300000000000002),
 .UNSPECIFIED.);
#844=B_SPLINE_SURFACE_WITH_KNOTS('',2,1,((#23756,#23757),(#23758,#23759),
(#23760,#23761)),.UNSPECIFIED.,.F.,.F.,.F.,(3,3),(2,2),(0.,1.),(0.,0.0300000000000002),
 .UNSPECIFIED.);
#845=B_SPLINE_SURFACE_WITH_KNOTS('',2,1,((#23767,#23768),(#23769,#23770),
(#23771,#23772)),.UNSPECIFIED.,.F.,.F.,.F.,(3,3),(2,2),(0.,1.),(0.,0.0300000000000002),
 .UNSPECIFIED.);
#846=B_SPLINE_SURFACE_WITH_KNOTS('',2,1,((#23778,#23779),(#23780,#23781),
(#23782,#23783)),.UNSPECIFIED.,.F.,.F.,.F.,(3,3),(2,2),(0.,1.),(0.,0.0300000000000002),
 .UNSPECIFIED.);
#847=B_SPLINE_SURFACE_WITH_KNOTS('',2,1,((#23789,#23790),(#23791,#23792),
(#23793,#23794)),.UNSPECIFIED.,.F.,.F.,.F.,(3,3),(2,2),(0.,1.),(0.,0.0300000000000002),
 .UNSPECIFIED.);
#848=B_SPLINE_SURFACE_WITH_KNOTS('',2,1,((#23800,#23801),(#23802,#23803),
(#23804,#23805)),.UNSPECIFIED.,.F.,.F.,.F.,(3,3),(2,2),(0.,1.),(0.,0.0300000000000002),
 .UNSPECIFIED.);
#849=B_SPLINE_SURFACE_WITH_KNOTS('',2,1,((#23811,#23812),(#23813,#23814),
(#23815,#23816)),.UNSPECIFIED.,.F.,.F.,.F.,(3,3),(2,2),(0.,1.),(0.,0.0300000000000002),
 .UNSPECIFIED.);
#850=B_SPLINE_SURFACE_WITH_KNOTS('',2,1,((#23822,#23823),(#23824,#23825),
(#23826,#23827)),.UNSPECIFIED.,.F.,.F.,.F.,(3,3),(2,2),(0.,1.),(0.,0.0300000000000002),
 .UNSPECIFIED.);
#851=B_SPLINE_SURFACE_WITH_KNOTS('',2,1,((#23833,#23834),(#23835,#23836),
(#23837,#23838)),.UNSPECIFIED.,.F.,.F.,.F.,(3,3),(2,2),(0.,1.),(0.,0.0300000000000002),
 .UNSPECIFIED.);
#852=B_SPLINE_SURFACE_WITH_KNOTS('',2,1,((#23844,#23845),(#23846,#23847),
(#23848,#23849)),.UNSPECIFIED.,.F.,.F.,.F.,(3,3),(2,2),(0.,1.),(0.,0.0300000000000002),
 .UNSPECIFIED.);
#939=FACE_BOUND('',#2792,.T.);
#940=FACE_BOUND('',#2795,.T.);
#941=FACE_BOUND('',#2847,.T.);
#942=FACE_BOUND('',#2848,.T.);
#943=FACE_BOUND('',#2849,.T.);
#944=FACE_BOUND('',#2850,.T.);
#945=FACE_BOUND('',#2877,.T.);
#946=FACE_BOUND('',#2892,.T.);
#1062=PLANE('',#16766);
#1063=PLANE('',#16770);
#1064=PLANE('',#16774);
#1065=PLANE('',#16776);
#1066=PLANE('',#16781);
#1067=PLANE('',#16783);
#1068=PLANE('',#16786);
#1069=PLANE('',#16789);
#1070=PLANE('',#16801);
#1071=PLANE('',#16855);
#1072=PLANE('',#16856);
#1073=PLANE('',#16861);
#1074=PLANE('',#16867);
#1075=PLANE('',#16869);
#1076=PLANE('',#16873);
#1077=PLANE('',#16885);
#1078=PLANE('',#16888);
#1079=PLANE('',#16898);
#1080=PLANE('',#16933);
#1081=PLANE('',#16936);
#1082=PLANE('',#16938);
#1083=PLANE('',#16939);
#1084=PLANE('',#16940);
#1085=PLANE('',#16941);
#1086=PLANE('',#16942);
#1087=PLANE('',#16943);
#1088=PLANE('',#16944);
#1089=PLANE('',#16945);
#1090=PLANE('',#16946);
#1091=PLANE('',#16947);
#1092=PLANE('',#16948);
#1093=PLANE('',#16949);
#1094=PLANE('',#16950);
#1095=PLANE('',#16951);
#1096=PLANE('',#16952);
#1097=PLANE('',#16953);
#1098=PLANE('',#16954);
#1099=PLANE('',#16955);
#1100=PLANE('',#16956);
#1101=PLANE('',#16957);
#1102=PLANE('',#16958);
#1103=PLANE('',#16959);
#1104=PLANE('',#16962);
#1105=PLANE('',#16966);
#1106=PLANE('',#16967);
#1107=PLANE('',#16968);
#1563=CYLINDRICAL_SURFACE('',#16764,15.2);
#1564=CYLINDRICAL_SURFACE('',#16779,1.5);
#1565=CYLINDRICAL_SURFACE('',#16784,1.5);
#1566=CYLINDRICAL_SURFACE('',#16787,1.5);
#1567=CYLINDRICAL_SURFACE('',#16790,1.5);
#1568=CYLINDRICAL_SURFACE('',#16799,1.5);
#1569=CYLINDRICAL_SURFACE('',#16800,1.5);
#1570=CYLINDRICAL_SURFACE('',#16806,1.5);
#1571=CYLINDRICAL_SURFACE('',#16807,1.5);
#1572=CYLINDRICAL_SURFACE('',#16815,1.5);
#1573=CYLINDRICAL_SURFACE('',#16816,1.5);
#1574=CYLINDRICAL_SURFACE('',#16825,1.5);
#1575=CYLINDRICAL_SURFACE('',#16826,1.5);
#1576=CYLINDRICAL_SURFACE('',#16834,1.5);
#1577=CYLINDRICAL_SURFACE('',#16835,1.5);
#1578=CYLINDRICAL_SURFACE('',#16840,1.5);
#1579=CYLINDRICAL_SURFACE('',#16845,1.5);
#1580=CYLINDRICAL_SURFACE('',#16847,1.5);
#1581=CYLINDRICAL_SURFACE('',#16852,1.5);
#1582=CYLINDRICAL_SURFACE('',#16857,1.5);
#1583=CYLINDRICAL_SURFACE('',#16858,1.5);
#1584=CYLINDRICAL_SURFACE('',#16859,1.5);
#1585=CYLINDRICAL_SURFACE('',#16862,1.5);
#1586=CYLINDRICAL_SURFACE('',#16863,1.5);
#1587=CYLINDRICAL_SURFACE('',#16865,1.5);
#1588=CYLINDRICAL_SURFACE('',#16866,1.5);
#1589=CYLINDRICAL_SURFACE('',#16871,1.5);
#1590=CYLINDRICAL_SURFACE('',#16872,1.5);
#1591=CYLINDRICAL_SURFACE('',#16878,1.5);
#1592=CYLINDRICAL_SURFACE('',#16879,1.5);
#1593=CYLINDRICAL_SURFACE('',#16884,1.5);
#1594=CYLINDRICAL_SURFACE('',#16886,1.5);
#1595=CYLINDRICAL_SURFACE('',#16887,1.5);
#1596=CYLINDRICAL_SURFACE('',#16904,27.);
#1597=CYLINDRICAL_SURFACE('',#16911,1.5);
#1598=CYLINDRICAL_SURFACE('',#16917,1.5);
#1599=CYLINDRICAL_SURFACE('',#16923,1.5);
#1600=CYLINDRICAL_SURFACE('',#16931,1.5);
#1601=CYLINDRICAL_SURFACE('',#16935,3.);
#1602=CYLINDRICAL_SURFACE('',#16937,3.);
#1603=CYLINDRICAL_SURFACE('',#16960,3.05);
#1604=CYLINDRICAL_SURFACE('',#16965,21.05);
#1815=FACE_OUTER_BOUND('',#2789,.T.);
#1816=FACE_OUTER_BOUND('',#2790,.T.);
#1817=FACE_OUTER_BOUND('',#2791,.T.);
#1818=FACE_OUTER_BOUND('',#2793,.T.);
#1819=FACE_OUTER_BOUND('',#2794,.T.);
#1820=FACE_OUTER_BOUND('',#2796,.T.);
#1821=FACE_OUTER_BOUND('',#2797,.T.);
#1822=FACE_OUTER_BOUND('',#2798,.T.);
#1823=FACE_OUTER_BOUND('',#2799,.T.);
#1824=FACE_OUTER_BOUND('',#2800,.T.);
#1825=FACE_OUTER_BOUND('',#2801,.T.);
#1826=FACE_OUTER_BOUND('',#2802,.T.);
#1827=FACE_OUTER_BOUND('',#2803,.T.);
#1828=FACE_OUTER_BOUND('',#2804,.T.);
#1829=FACE_OUTER_BOUND('',#2805,.T.);
#1830=FACE_OUTER_BOUND('',#2806,.T.);
#1831=FACE_OUTER_BOUND('',#2807,.T.);
#1832=FACE_OUTER_BOUND('',#2808,.T.);
#1833=FACE_OUTER_BOUND('',#2809,.T.);
#1834=FACE_OUTER_BOUND('',#2810,.T.);
#1835=FACE_OUTER_BOUND('',#2811,.T.);
#1836=FACE_OUTER_BOUND('',#2812,.T.);
#1837=FACE_OUTER_BOUND('',#2813,.T.);
#1838=FACE_OUTER_BOUND('',#2814,.T.);
#1839=FACE_OUTER_BOUND('',#2815,.T.);
#1840=FACE_OUTER_BOUND('',#2816,.T.);
#1841=FACE_OUTER_BOUND('',#2817,.T.);
#1842=FACE_OUTER_BOUND('',#2818,.T.);
#1843=FACE_OUTER_BOUND('',#2819,.T.);
#1844=FACE_OUTER_BOUND('',#2820,.T.);
#1845=FACE_OUTER_BOUND('',#2821,.T.);
#1846=FACE_OUTER_BOUND('',#2822,.T.);
#1847=FACE_OUTER_BOUND('',#2823,.T.);
#1848=FACE_OUTER_BOUND('',#2824,.T.);
#1849=FACE_OUTER_BOUND('',#2825,.T.);
#1850=FACE_OUTER_BOUND('',#2826,.T.);
#1851=FACE_OUTER_BOUND('',#2827,.T.);
#1852=FACE_OUTER_BOUND('',#2828,.T.);
#1853=FACE_OUTER_BOUND('',#2829,.T.);
#1854=FACE_OUTER_BOUND('',#2830,.T.);
#1855=FACE_OUTER_BOUND('',#2831,.T.);
#1856=FACE_OUTER_BOUND('',#2832,.T.);
#1857=FACE_OUTER_BOUND('',#2833,.T.);
#1858=FACE_OUTER_BOUND('',#2834,.T.);
#1859=FACE_OUTER_BOUND('',#2835,.T.);
#1860=FACE_OUTER_BOUND('',#2836,.T.);
#1861=FACE_OUTER_BOUND('',#2837,.T.);
#1862=FACE_OUTER_BOUND('',#2838,.T.);
#1863=FACE_OUTER_BOUND('',#2839,.T.);
#1864=FACE_OUTER_BOUND('',#2840,.T.);
#1865=FACE_OUTER_BOUND('',#2841,.T.);
#1866=FACE_OUTER_BOUND('',#2842,.T.);
#1867=FACE_OUTER_BOUND('',#2843,.T.);
#1868=FACE_OUTER_BOUND('',#2844,.T.);
#1869=FACE_OUTER_BOUND('',#2845,.T.);
#1870=FACE_OUTER_BOUND('',#2846,.T.);
#1871=FACE_OUTER_BOUND('',#2851,.T.);
#1872=FACE_OUTER_BOUND('',#2852,.T.);
#1873=FACE_OUTER_BOUND('',#2853,.T.);
#1874=FACE_OUTER_BOUND('',#2854,.T.);
#1875=FACE_OUTER_BOUND('',#2855,.T.);
#1876=FACE_OUTER_BOUND('',#2856,.T.);
#1877=FACE_OUTER_BOUND('',#2857,.T.);
#1878=FACE_OUTER_BOUND('',#2858,.T.);
#1879=FACE_OUTER_BOUND('',#2859,.T.);
#1880=FACE_OUTER_BOUND('',#2860,.T.);
#1881=FACE_OUTER_BOUND('',#2861,.T.);
#1882=FACE_OUTER_BOUND('',#2862,.T.);
#1883=FACE_OUTER_BOUND('',#2863,.T.);
#1884=FACE_OUTER_BOUND('',#2864,.T.);
#1885=FACE_OUTER_BOUND('',#2865,.T.);
#1886=FACE_OUTER_BOUND('',#2866,.T.);
#1887=FACE_OUTER_BOUND('',#2867,.T.);
#1888=FACE_OUTER_BOUND('',#2868,.T.);
#1889=FACE_OUTER_BOUND('',#2869,.T.);
#1890=FACE_OUTER_BOUND('',#2870,.T.);
#1891=FACE_OUTER_BOUND('',#2871,.T.);
#1892=FACE_OUTER_BOUND('',#2872,.T.);
#1893=FACE_OUTER_BOUND('',#2873,.T.);
#1894=FACE_OUTER_BOUND('',#2874,.T.);
#1895=FACE_OUTER_BOUND('',#2875,.T.);
#1896=FACE_OUTER_BOUND('',#2876,.T.);
#1897=FACE_OUTER_BOUND('',#2878,.T.);
#1898=FACE_OUTER_BOUND('',#2879,.T.);
#1899=FACE_OUTER_BOUND('',#2880,.T.);
#1900=FACE_OUTER_BOUND('',#2881,.T.);
#1901=FACE_OUTER_BOUND('',#2882,.T.);
#1902=FACE_OUTER_BOUND('',#2883,.T.);
#1903=FACE_OUTER_BOUND('',#2884,.T.);
#1904=FACE_OUTER_BOUND('',#2885,.T.);
#1905=FACE_OUTER_BOUND('',#2886,.T.);
#1906=FACE_OUTER_BOUND('',#2887,.T.);
#1907=FACE_OUTER_BOUND('',#2888,.T.);
#1908=FACE_OUTER_BOUND('',#2889,.T.);
#1909=FACE_OUTER_BOUND('',#2890,.T.);
#1910=FACE_OUTER_BOUND('',#2891,.T.);
#1911=FACE_OUTER_BOUND('',#2893,.T.);
#1912=FACE_OUTER_BOUND('',#2894,.T.);
#1913=FACE_OUTER_BOUND('',#2895,.T.);
#1914=FACE_OUTER_BOUND('',#2896,.T.);
#1915=FACE_OUTER_BOUND('',#2897,.T.);
#1916=FACE_OUTER_BOUND('',#2898,.T.);
#1917=FACE_OUTER_BOUND('',#2899,.T.);
#1918=FACE_OUTER_BOUND('',#2900,.T.);
#1919=FACE_OUTER_BOUND('',#2901,.T.);
#1920=FACE_OUTER_BOUND('',#2902,.T.);
#1921=FACE_OUTER_BOUND('',#2903,.T.);
#1922=FACE_OUTER_BOUND('',#2904,.T.);
#1923=FACE_OUTER_BOUND('',#2905,.T.);
#1924=FACE_OUTER_BOUND('',#2906,.T.);
#1925=FACE_OUTER_BOUND('',#2907,.T.);
#1926=FACE_OUTER_BOUND('',#2908,.T.);
#1927=FACE_OUTER_BOUND('',#2909,.T.);
#1928=FACE_OUTER_BOUND('',#2910,.T.);
#1929=FACE_OUTER_BOUND('',#2911,.T.);
#1930=FACE_OUTER_BOUND('',#2912,.T.);
#1931=FACE_OUTER_BOUND('',#2913,.T.);
#1932=FACE_OUTER_BOUND('',#2914,.T.);
#1933=FACE_OUTER_BOUND('',#2915,.T.);
#1934=FACE_OUTER_BOUND('',#2916,.T.);
#1935=FACE_OUTER_BOUND('',#2917,.T.);
#1936=FACE_OUTER_BOUND('',#2918,.T.);
#1937=FACE_OUTER_BOUND('',#2919,.T.);
#1938=FACE_OUTER_BOUND('',#2920,.T.);
#1939=FACE_OUTER_BOUND('',#2921,.T.);
#1940=FACE_OUTER_BOUND('',#2922,.T.);
#1941=FACE_OUTER_BOUND('',#2923,.T.);
#1942=FACE_OUTER_BOUND('',#2924,.T.);
#1943=FACE_OUTER_BOUND('',#2925,.T.);
#1944=FACE_OUTER_BOUND('',#2926,.T.);
#1945=FACE_OUTER_BOUND('',#2927,.T.);
#1946=FACE_OUTER_BOUND('',#2928,.T.);
#1947=FACE_OUTER_BOUND('',#2929,.T.);
#1948=FACE_OUTER_BOUND('',#2930,.T.);
#1949=FACE_OUTER_BOUND('',#2931,.T.);
#1950=FACE_OUTER_BOUND('',#2932,.T.);
#1951=FACE_OUTER_BOUND('',#2933,.T.);
#1952=FACE_OUTER_BOUND('',#2934,.T.);
#1953=FACE_OUTER_BOUND('',#2935,.T.);
#1954=FACE_OUTER_BOUND('',#2936,.T.);
#1955=FACE_OUTER_BOUND('',#2937,.T.);
#1956=FACE_OUTER_BOUND('',#2938,.T.);
#1957=FACE_OUTER_BOUND('',#2939,.T.);
#1958=FACE_OUTER_BOUND('',#2940,.T.);
#1959=FACE_OUTER_BOUND('',#2941,.T.);
#1960=FACE_OUTER_BOUND('',#2942,.T.);
#1961=FACE_OUTER_BOUND('',#2943,.T.);
#1962=FACE_OUTER_BOUND('',#2944,.T.);
#1963=FACE_OUTER_BOUND('',#2945,.T.);
#1964=FACE_OUTER_BOUND('',#2946,.T.);
#1965=FACE_OUTER_BOUND('',#2947,.T.);
#1966=FACE_OUTER_BOUND('',#2948,.T.);
#1967=FACE_OUTER_BOUND('',#2949,.T.);
#1968=FACE_OUTER_BOUND('',#2950,.T.);
#1969=FACE_OUTER_BOUND('',#2951,.T.);
#2789=EDGE_LOOP('',(#10802,#10803,#10804,#10805,#10806));
#2790=EDGE_LOOP('',(#10807,#10808,#10809,#10810,#10811));
#2791=EDGE_LOOP('',(#10812));
#2792=EDGE_LOOP('',(#10813));
#2793=EDGE_LOOP('',(#10814,#10815,#10816,#10817));
#2794=EDGE_LOOP('',(#10818,#10819,#10820,#10821,#10822,#10823,#10824,#10825,
#10826,#10827));
#2795=EDGE_LOOP('',(#10828));
#2796=EDGE_LOOP('',(#10829,#10830,#10831,#10832));
#2797=EDGE_LOOP('',(#10833,#10834,#10835,#10836));
#2798=EDGE_LOOP('',(#10837,#10838,#10839,#10840));
#2799=EDGE_LOOP('',(#10841,#10842,#10843,#10844,#10845,#10846,#10847,#10848,
#10849,#10850,#10851,#10852,#10853,#10854));
#2800=EDGE_LOOP('',(#10855,#10856,#10857,#10858,#10859));
#2801=EDGE_LOOP('',(#10860,#10861,#10862,#10863,#10864,#10865));
#2802=EDGE_LOOP('',(#10866,#10867,#10868,#10869));
#2803=EDGE_LOOP('',(#10870,#10871,#10872,#10873));
#2804=EDGE_LOOP('',(#10874,#10875,#10876,#10877));
#2805=EDGE_LOOP('',(#10878,#10879,#10880,#10881));
#2806=EDGE_LOOP('',(#10882,#10883,#10884,#10885));
#2807=EDGE_LOOP('',(#10886,#10887,#10888,#10889));
#2808=EDGE_LOOP('',(#10890,#10891,#10892,#10893));
#2809=EDGE_LOOP('',(#10894,#10895,#10896,#10897));
#2810=EDGE_LOOP('',(#10898,#10899,#10900,#10901));
#2811=EDGE_LOOP('',(#10902,#10903,#10904,#10905));
#2812=EDGE_LOOP('',(#10906,#10907,#10908,#10909));
#2813=EDGE_LOOP('',(#10910,#10911,#10912,#10913,#10914,#10915,#10916));
#2814=EDGE_LOOP('',(#10917,#10918,#10919,#10920,#10921));
#2815=EDGE_LOOP('',(#10922,#10923,#10924,#10925,#10926));
#2816=EDGE_LOOP('',(#10927,#10928,#10929,#10930,#10931,#10932,#10933,#10934,
#10935,#10936));
#2817=EDGE_LOOP('',(#10937,#10938,#10939,#10940));
#2818=EDGE_LOOP('',(#10941,#10942,#10943));
#2819=EDGE_LOOP('',(#10944,#10945,#10946));
#2820=EDGE_LOOP('',(#10947,#10948,#10949,#10950));
#2821=EDGE_LOOP('',(#10951,#10952,#10953,#10954));
#2822=EDGE_LOOP('',(#10955,#10956,#10957,#10958));
#2823=EDGE_LOOP('',(#10959,#10960,#10961));
#2824=EDGE_LOOP('',(#10962,#10963,#10964,#10965));
#2825=EDGE_LOOP('',(#10966,#10967,#10968,#10969));
#2826=EDGE_LOOP('',(#10970,#10971,#10972));
#2827=EDGE_LOOP('',(#10973,#10974,#10975));
#2828=EDGE_LOOP('',(#10976,#10977,#10978,#10979));
#2829=EDGE_LOOP('',(#10980,#10981,#10982,#10983));
#2830=EDGE_LOOP('',(#10984,#10985,#10986));
#2831=EDGE_LOOP('',(#10987,#10988,#10989));
#2832=EDGE_LOOP('',(#10990,#10991,#10992,#10993));
#2833=EDGE_LOOP('',(#10994,#10995,#10996,#10997));
#2834=EDGE_LOOP('',(#10998,#10999,#11000));
#2835=EDGE_LOOP('',(#11001,#11002,#11003));
#2836=EDGE_LOOP('',(#11004,#11005,#11006,#11007));
#2837=EDGE_LOOP('',(#11008,#11009,#11010,#11011));
#2838=EDGE_LOOP('',(#11012,#11013,#11014));
#2839=EDGE_LOOP('',(#11015,#11016,#11017,#11018));
#2840=EDGE_LOOP('',(#11019,#11020,#11021));
#2841=EDGE_LOOP('',(#11022,#11023,#11024,#11025));
#2842=EDGE_LOOP('',(#11026,#11027,#11028,#11029,#11030));
#2843=EDGE_LOOP('',(#11031,#11032,#11033));
#2844=EDGE_LOOP('',(#11034,#11035,#11036,#11037,#11038,#11039,#11040));
#2845=EDGE_LOOP('',(#11041,#11042,#11043));
#2846=EDGE_LOOP('',(#11044,#11045,#11046,#11047));
#2847=EDGE_LOOP('',(#11048,#11049,#11050,#11051,#11052,#11053,#11054,#11055,
#11056,#11057,#11058));
#2848=EDGE_LOOP('',(#11059,#11060,#11061,#11062,#11063,#11064,#11065,#11066));
#2849=EDGE_LOOP('',(#11067,#11068,#11069,#11070,#11071,#11072,#11073,#11074,
#11075,#11076,#11077,#11078,#11079,#11080,#11081,#11082));
#2850=EDGE_LOOP('',(#11083,#11084,#11085,#11086,#11087,#11088,#11089,#11090,
#11091,#11092));
#2851=EDGE_LOOP('',(#11093,#11094,#11095,#11096));
#2852=EDGE_LOOP('',(#11097,#11098,#11099,#11100));
#2853=EDGE_LOOP('',(#11101,#11102,#11103,#11104));
#2854=EDGE_LOOP('',(#11105,#11106,#11107,#11108));
#2855=EDGE_LOOP('',(#11109,#11110,#11111,#11112,#11113));
#2856=EDGE_LOOP('',(#11114,#11115,#11116,#11117));
#2857=EDGE_LOOP('',(#11118,#11119,#11120,#11121));
#2858=EDGE_LOOP('',(#11122,#11123,#11124,#11125));
#2859=EDGE_LOOP('',(#11126,#11127,#11128,#11129,#11130));
#2860=EDGE_LOOP('',(#11131,#11132,#11133));
#2861=EDGE_LOOP('',(#11134,#11135,#11136));
#2862=EDGE_LOOP('',(#11137,#11138,#11139,#11140));
#2863=EDGE_LOOP('',(#11141,#11142,#11143,#11144));
#2864=EDGE_LOOP('',(#11145,#11146,#11147,#11148));
#2865=EDGE_LOOP('',(#11149,#11150,#11151));
#2866=EDGE_LOOP('',(#11152,#11153,#11154,#11155));
#2867=EDGE_LOOP('',(#11156,#11157,#11158,#11159));
#2868=EDGE_LOOP('',(#11160,#11161,#11162));
#2869=EDGE_LOOP('',(#11163,#11164,#11165,#11166));
#2870=EDGE_LOOP('',(#11167,#11168,#11169,#11170));
#2871=EDGE_LOOP('',(#11171,#11172,#11173,#11174));
#2872=EDGE_LOOP('',(#11175,#11176,#11177,#11178));
#2873=EDGE_LOOP('',(#11179,#11180,#11181));
#2874=EDGE_LOOP('',(#11182,#11183,#11184,#11185,#11186));
#2875=EDGE_LOOP('',(#11187,#11188,#11189,#11190,#11191,#11192));
#2876=EDGE_LOOP('',(#11193));
#2877=EDGE_LOOP('',(#11194));
#2878=EDGE_LOOP('',(#11195,#11196,#11197,#11198,#11199,#11200));
#2879=EDGE_LOOP('',(#11201,#11202,#11203,#11204,#11205,#11206,#11207,#11208,
#11209,#11210,#11211,#11212,#11213,#11214,#11215,#11216,#11217,#11218,#11219,
#11220,#11221,#11222,#11223,#11224,#11225,#11226,#11227));
#2880=EDGE_LOOP('',(#11228,#11229,#11230,#11231));
#2881=EDGE_LOOP('',(#11232,#11233,#11234,#11235));
#2882=EDGE_LOOP('',(#11236,#11237,#11238,#11239));
#2883=EDGE_LOOP('',(#11240,#11241,#11242,#11243));
#2884=EDGE_LOOP('',(#11244,#11245,#11246,#11247));
#2885=EDGE_LOOP('',(#11248,#11249,#11250,#11251));
#2886=EDGE_LOOP('',(#11252,#11253,#11254,#11255));
#2887=EDGE_LOOP('',(#11256,#11257,#11258,#11259,#11260));
#2888=EDGE_LOOP('',(#11261,#11262,#11263,#11264));
#2889=EDGE_LOOP('',(#11265,#11266,#11267,#11268));
#2890=EDGE_LOOP('',(#11269,#11270,#11271,#11272));
#2891=EDGE_LOOP('',(#11273,#11274,#11275,#11276));
#2892=EDGE_LOOP('',(#11277));
#2893=EDGE_LOOP('',(#11278,#11279,#11280,#11281));
#2894=EDGE_LOOP('',(#11282,#11283,#11284,#11285));
#2895=EDGE_LOOP('',(#11286,#11287,#11288,#11289));
#2896=EDGE_LOOP('',(#11290,#11291,#11292,#11293));
#2897=EDGE_LOOP('',(#11294,#11295,#11296,#11297));
#2898=EDGE_LOOP('',(#11298,#11299,#11300,#11301));
#2899=EDGE_LOOP('',(#11302,#11303,#11304,#11305));
#2900=EDGE_LOOP('',(#11306,#11307,#11308,#11309));
#2901=EDGE_LOOP('',(#11310,#11311,#11312,#11313));
#2902=EDGE_LOOP('',(#11314,#11315,#11316,#11317));
#2903=EDGE_LOOP('',(#11318,#11319,#11320,#11321));
#2904=EDGE_LOOP('',(#11322,#11323,#11324,#11325));
#2905=EDGE_LOOP('',(#11326,#11327,#11328,#11329));
#2906=EDGE_LOOP('',(#11330,#11331,#11332,#11333));
#2907=EDGE_LOOP('',(#11334,#11335,#11336,#11337,#11338,#11339,#11340,#11341,
#11342,#11343,#11344));
#2908=EDGE_LOOP('',(#11345,#11346,#11347,#11348));
#2909=EDGE_LOOP('',(#11349,#11350,#11351,#11352));
#2910=EDGE_LOOP('',(#11353,#11354,#11355,#11356));
#2911=EDGE_LOOP('',(#11357,#11358,#11359,#11360));
#2912=EDGE_LOOP('',(#11361,#11362,#11363,#11364));
#2913=EDGE_LOOP('',(#11365,#11366,#11367,#11368));
#2914=EDGE_LOOP('',(#11369,#11370,#11371,#11372));
#2915=EDGE_LOOP('',(#11373,#11374,#11375,#11376));
#2916=EDGE_LOOP('',(#11377,#11378,#11379,#11380,#11381,#11382,#11383,#11384));
#2917=EDGE_LOOP('',(#11385,#11386,#11387,#11388));
#2918=EDGE_LOOP('',(#11389,#11390,#11391,#11392));
#2919=EDGE_LOOP('',(#11393,#11394,#11395,#11396));
#2920=EDGE_LOOP('',(#11397,#11398,#11399,#11400));
#2921=EDGE_LOOP('',(#11401,#11402,#11403,#11404));
#2922=EDGE_LOOP('',(#11405,#11406,#11407,#11408));
#2923=EDGE_LOOP('',(#11409,#11410,#11411,#11412));
#2924=EDGE_LOOP('',(#11413,#11414,#11415,#11416));
#2925=EDGE_LOOP('',(#11417,#11418,#11419,#11420));
#2926=EDGE_LOOP('',(#11421,#11422,#11423,#11424));
#2927=EDGE_LOOP('',(#11425,#11426,#11427,#11428));
#2928=EDGE_LOOP('',(#11429,#11430,#11431,#11432));
#2929=EDGE_LOOP('',(#11433,#11434,#11435,#11436));
#2930=EDGE_LOOP('',(#11437,#11438,#11439,#11440));
#2931=EDGE_LOOP('',(#11441,#11442,#11443,#11444));
#2932=EDGE_LOOP('',(#11445,#11446,#11447,#11448));
#2933=EDGE_LOOP('',(#11449,#11450,#11451,#11452,#11453,#11454,#11455,#11456,
#11457,#11458,#11459,#11460,#11461,#11462,#11463,#11464));
#2934=EDGE_LOOP('',(#11465,#11466,#11467,#11468));
#2935=EDGE_LOOP('',(#11469,#11470,#11471,#11472));
#2936=EDGE_LOOP('',(#11473,#11474,#11475,#11476));
#2937=EDGE_LOOP('',(#11477,#11478,#11479,#11480));
#2938=EDGE_LOOP('',(#11481,#11482,#11483,#11484));
#2939=EDGE_LOOP('',(#11485,#11486,#11487,#11488));
#2940=EDGE_LOOP('',(#11489,#11490,#11491,#11492));
#2941=EDGE_LOOP('',(#11493,#11494,#11495,#11496));
#2942=EDGE_LOOP('',(#11497,#11498,#11499,#11500));
#2943=EDGE_LOOP('',(#11501,#11502,#11503,#11504));
#2944=EDGE_LOOP('',(#11505,#11506,#11507,#11508,#11509,#11510,#11511,#11512,
#11513,#11514));
#2945=EDGE_LOOP('',(#11515,#11516,#11517,#11518));
#2946=EDGE_LOOP('',(#11519));
#2947=EDGE_LOOP('',(#11520,#11521,#11522,#11523));
#2948=EDGE_LOOP('',(#11524,#11525,#11526,#11527));
#2949=EDGE_LOOP('',(#11528,#11529,#11530,#11531,#11532,#11533,#11534,#11535,
#11536,#11537,#11538,#11539,#11540,#11541,#11542));
#2950=EDGE_LOOP('',(#11543,#11544,#11545));
#2951=EDGE_LOOP('',(#11546,#11547,#11548,#11549));
#3886=LINE('',#22172,#5197);
#3887=LINE('',#22177,#5198);
#3888=LINE('',#22184,#5199);
#3889=LINE('',#22190,#5200);
#3890=LINE('',#22192,#5201);
#3891=LINE('',#22194,#5202);
#3892=LINE('',#22198,#5203);
#3893=LINE('',#22200,#5204);
#3894=LINE('',#22204,#5205);
#3895=LINE('',#22205,#5206);
#3896=LINE('',#22348,#5207);
#3897=LINE('',#22376,#5208);
#3898=LINE('',#22386,#5209);
#3899=LINE('',#22387,#5210);
#3900=LINE('',#22390,#5211);
#3901=LINE('',#22392,#5212);
#3902=LINE('',#22394,#5213);
#3903=LINE('',#22396,#5214);
#3904=LINE('',#22398,#5215);
#3905=LINE('',#22400,#5216);
#3906=LINE('',#22402,#5217);
#3907=LINE('',#22406,#5218);
#3908=LINE('',#22410,#5219);
#3909=LINE('',#22412,#5220);
#3910=LINE('',#22413,#5221);
#3911=LINE('',#22416,#5222);
#3912=LINE('',#22422,#5223);
#3913=LINE('',#22424,#5224);
#3914=LINE('',#22425,#5225);
#3915=LINE('',#22568,#5226);
#3916=LINE('',#22711,#5227);
#3917=LINE('',#22734,#5228);
#3918=LINE('',#22757,#5229);
#3919=LINE('',#22764,#5230);
#3920=LINE('',#22796,#5231);
#3921=LINE('',#22798,#5232);
#3922=LINE('',#22800,#5233);
#3923=LINE('',#22801,#5234);
#3924=LINE('',#22844,#5235);
#3925=LINE('',#22851,#5236);
#3926=LINE('',#22902,#5237);
#3927=LINE('',#22933,#5238);
#3928=LINE('',#22936,#5239);
#3929=LINE('',#22939,#5240);
#3930=LINE('',#22941,#5241);
#3931=LINE('',#22942,#5242);
#3932=LINE('',#22945,#5243);
#3933=LINE('',#22949,#5244);
#3934=LINE('',#22950,#5245);
#3935=LINE('',#22956,#5246);
#3936=LINE('',#22959,#5247);
#3937=LINE('',#22969,#5248);
#3938=LINE('',#22983,#5249);
#3939=LINE('',#22986,#5250);
#3940=LINE('',#22998,#5251);
#3941=LINE('',#23001,#5252);
#3942=LINE('',#23002,#5253);
#3943=LINE('',#23019,#5254);
#3944=LINE('',#23035,#5255);
#3945=LINE('',#23036,#5256);
#3946=LINE('',#23048,#5257);
#3947=LINE('',#23050,#5258);
#3948=LINE('',#23065,#5259);
#3949=LINE('',#23066,#5260);
#3950=LINE('',#23068,#5261);
#3951=LINE('',#23069,#5262);
#3952=LINE('',#23080,#5263);
#3953=LINE('',#23082,#5264);
#3954=LINE('',#23083,#5265);
#3955=LINE('',#23092,#5266);
#3956=LINE('',#23100,#5267);
#3957=LINE('',#23109,#5268);
#3958=LINE('',#23110,#5269);
#3959=LINE('',#23114,#5270);
#3960=LINE('',#23161,#5271);
#3961=LINE('',#23163,#5272);
#3962=LINE('',#23165,#5273);
#3963=LINE('',#23167,#5274);
#3964=LINE('',#23169,#5275);
#3965=LINE('',#23171,#5276);
#3966=LINE('',#23173,#5277);
#3967=LINE('',#23174,#5278);
#3968=LINE('',#23241,#5279);
#3969=LINE('',#23243,#5280);
#3970=LINE('',#23245,#5281);
#3971=LINE('',#23247,#5282);
#3972=LINE('',#23249,#5283);
#3973=LINE('',#23251,#5284);
#3974=LINE('',#23253,#5285);
#3975=LINE('',#23255,#5286);
#3976=LINE('',#23257,#5287);
#3977=LINE('',#23258,#5288);
#3978=LINE('',#23260,#5289);
#3979=LINE('',#23265,#5290);
#3980=LINE('',#23268,#5291);
#3981=LINE('',#23270,#5292);
#3982=LINE('',#23273,#5293);
#3983=LINE('',#23276,#5294);
#3984=LINE('',#23292,#5295);
#3985=LINE('',#23299,#5296);
#3986=LINE('',#23330,#5297);
#3987=LINE('',#23353,#5298);
#3988=LINE('',#23370,#5299);
#3989=LINE('',#23379,#5300);
#3990=LINE('',#23380,#5301);
#3991=LINE('',#23383,#5302);
#3992=LINE('',#23384,#5303);
#3993=LINE('',#23387,#5304);
#3994=LINE('',#23400,#5305);
#3995=LINE('',#23414,#5306);
#3996=LINE('',#23427,#5307);
#3997=LINE('',#23442,#5308);
#3998=LINE('',#23445,#5309);
#3999=LINE('',#23448,#5310);
#4000=LINE('',#23457,#5311);
#4001=LINE('',#23460,#5312);
#4002=LINE('',#23468,#5313);
#4003=LINE('',#23497,#5314);
#4004=LINE('',#23514,#5315);
#4005=LINE('',#23518,#5316);
#4006=LINE('',#23520,#5317);
#4007=LINE('',#23529,#5318);
#4008=LINE('',#23534,#5319);
#4009=LINE('',#23542,#5320);
#4010=LINE('',#23553,#5321);
#4011=LINE('',#23564,#5322);
#4012=LINE('',#23575,#5323);
#4013=LINE('',#23586,#5324);
#4014=LINE('',#23597,#5325);
#4015=LINE('',#23608,#5326);
#4016=LINE('',#23619,#5327);
#4017=LINE('',#23630,#5328);
#4018=LINE('',#23646,#5329);
#4019=LINE('',#23648,#5330);
#4020=LINE('',#23649,#5331);
#4021=LINE('',#23652,#5332);
#4022=LINE('',#23653,#5333);
#4023=LINE('',#23656,#5334);
#4024=LINE('',#23657,#5335);
#4025=LINE('',#23660,#5336);
#4026=LINE('',#23661,#5337);
#4027=LINE('',#23664,#5338);
#4028=LINE('',#23665,#5339);
#4029=LINE('',#23668,#5340);
#4030=LINE('',#23669,#5341);
#4031=LINE('',#23672,#5342);
#4032=LINE('',#23673,#5343);
#4033=LINE('',#23675,#5344);
#4034=LINE('',#23684,#5345);
#4035=LINE('',#23689,#5346);
#4036=LINE('',#23697,#5347);
#4037=LINE('',#23708,#5348);
#4038=LINE('',#23719,#5349);
#4039=LINE('',#23730,#5350);
#4040=LINE('',#23741,#5351);
#4041=LINE('',#23752,#5352);
#4042=LINE('',#23763,#5353);
#4043=LINE('',#23774,#5354);
#4044=LINE('',#23785,#5355);
#4045=LINE('',#23796,#5356);
#4046=LINE('',#23807,#5357);
#4047=LINE('',#23818,#5358);
#4048=LINE('',#23829,#5359);
#4049=LINE('',#23840,#5360);
#4050=LINE('',#23856,#5361);
#4051=LINE('',#23858,#5362);
#4052=LINE('',#23859,#5363);
#4053=LINE('',#23862,#5364);
#4054=LINE('',#23863,#5365);
#4055=LINE('',#23866,#5366);
#4056=LINE('',#23867,#5367);
#4057=LINE('',#23870,#5368);
#4058=LINE('',#23871,#5369);
#4059=LINE('',#23874,#5370);
#4060=LINE('',#23875,#5371);
#4061=LINE('',#23878,#5372);
#4062=LINE('',#23879,#5373);
#4063=LINE('',#23882,#5374);
#4064=LINE('',#23883,#5375);
#4065=LINE('',#23886,#5376);
#4066=LINE('',#23887,#5377);
#4067=LINE('',#23890,#5378);
#4068=LINE('',#23891,#5379);
#4069=LINE('',#23893,#5380);
#4070=LINE('',#23897,#5381);
#4071=LINE('',#23903,#5382);
#4072=LINE('',#23905,#5383);
#5197=VECTOR('',#18133,15.45);
#5198=VECTOR('',#18140,15.2);
#5199=VECTOR('',#18149,15.45);
#5200=VECTOR('',#18154,10.);
#5201=VECTOR('',#18155,10.);
#5202=VECTOR('',#18156,10.);
#5203=VECTOR('',#18159,10.);
#5204=VECTOR('',#18160,10.);
#5205=VECTOR('',#18163,10.);
#5206=VECTOR('',#18164,10.);
#5207=VECTOR('',#18165,10.);
#5208=VECTOR('',#18166,10.);
#5209=VECTOR('',#18171,10.);
#5210=VECTOR('',#18172,10.);
#5211=VECTOR('',#18175,10.);
#5212=VECTOR('',#18176,10.);
#5213=VECTOR('',#18177,10.);
#5214=VECTOR('',#18178,10.);
#5215=VECTOR('',#18179,10.);
#5216=VECTOR('',#18180,10.);
#5217=VECTOR('',#18181,10.);
#5218=VECTOR('',#18184,10.);
#5219=VECTOR('',#18187,10.);
#5220=VECTOR('',#18188,10.);
#5221=VECTOR('',#18189,10.);
#5222=VECTOR('',#18192,10.);
#5223=VECTOR('',#18199,10.);
#5224=VECTOR('',#18200,10.);
#5225=VECTOR('',#18201,10.);
#5226=VECTOR('',#18202,10.);
#5227=VECTOR('',#18203,10.);
#5228=VECTOR('',#18204,10.);
#5229=VECTOR('',#18205,10.);
#5230=VECTOR('',#18206,10.);
#5231=VECTOR('',#18209,10.);
#5232=VECTOR('',#18210,10.);
#5233=VECTOR('',#18211,10.);
#5234=VECTOR('',#18212,10.);
#5235=VECTOR('',#18213,10.);
#5236=VECTOR('',#18214,10.);
#5237=VECTOR('',#18215,10.);
#5238=VECTOR('',#18218,10.);
#5239=VECTOR('',#18221,10.);
#5240=VECTOR('',#18224,10.);
#5241=VECTOR('',#18225,10.);
#5242=VECTOR('',#18226,10.);
#5243=VECTOR('',#18229,10.);
#5244=VECTOR('',#18234,10.);
#5245=VECTOR('',#18235,10.);
#5246=VECTOR('',#18240,10.);
#5247=VECTOR('',#18243,10.);
#5248=VECTOR('',#18258,10.);
#5249=VECTOR('',#18259,10.);
#5250=VECTOR('',#18262,10.);
#5251=VECTOR('',#18263,10.);
#5252=VECTOR('',#18266,10.);
#5253=VECTOR('',#18267,10.);
#5254=VECTOR('',#18278,10.);
#5255=VECTOR('',#18281,10.);
#5256=VECTOR('',#18282,10.);
#5257=VECTOR('',#18299,10.);
#5258=VECTOR('',#18302,10.);
#5259=VECTOR('',#18321,10.);
#5260=VECTOR('',#18322,10.);
#5261=VECTOR('',#18325,10.);
#5262=VECTOR('',#18326,10.);
#5263=VECTOR('',#18343,10.);
#5264=VECTOR('',#18346,10.);
#5265=VECTOR('',#18347,10.);
#5266=VECTOR('',#18360,10.);
#5267=VECTOR('',#18373,10.);
#5268=VECTOR('',#18384,10.);
#5269=VECTOR('',#18385,10.);
#5270=VECTOR('',#18392,10.);
#5271=VECTOR('',#18393,10.);
#5272=VECTOR('',#18394,10.);
#5273=VECTOR('',#18395,10.);
#5274=VECTOR('',#18396,10.);
#5275=VECTOR('',#18397,10.);
#5276=VECTOR('',#18398,10.);
#5277=VECTOR('',#18399,10.);
#5278=VECTOR('',#18400,10.);
#5279=VECTOR('',#18401,10.);
#5280=VECTOR('',#18402,10.);
#5281=VECTOR('',#18403,10.);
#5282=VECTOR('',#18404,10.);
#5283=VECTOR('',#18405,10.);
#5284=VECTOR('',#18406,10.);
#5285=VECTOR('',#18407,10.);
#5286=VECTOR('',#18408,10.);
#5287=VECTOR('',#18409,10.);
#5288=VECTOR('',#18410,10.);
#5289=VECTOR('',#18413,10.);
#5290=VECTOR('',#18420,10.);
#5291=VECTOR('',#18425,10.);
#5292=VECTOR('',#18428,10.);
#5293=VECTOR('',#18431,10.);
#5294=VECTOR('',#18434,10.);
#5295=VECTOR('',#18439,10.);
#5296=VECTOR('',#18450,10.);
#5297=VECTOR('',#18455,10.);
#5298=VECTOR('',#18466,10.);
#5299=VECTOR('',#18469,10.);
#5300=VECTOR('',#18480,10.);
#5301=VECTOR('',#18481,10.);
#5302=VECTOR('',#18484,10.);
#5303=VECTOR('',#18485,10.);
#5304=VECTOR('',#18488,10.);
#5305=VECTOR('',#18491,10.);
#5306=VECTOR('',#18492,10.);
#5307=VECTOR('',#18509,26.5);
#5308=VECTOR('',#18528,27.);
#5309=VECTOR('',#18533,10.);
#5310=VECTOR('',#18536,10.);
#5311=VECTOR('',#18547,10.);
#5312=VECTOR('',#18550,10.);
#5313=VECTOR('',#18561,10.);
#5314=VECTOR('',#18588,10.);
#5315=VECTOR('',#18593,10.);
#5316=VECTOR('',#18598,10.);
#5317=VECTOR('',#18601,10.);
#5318=VECTOR('',#18604,10.);
#5319=VECTOR('',#18605,10.);
#5320=VECTOR('',#18606,10.);
#5321=VECTOR('',#18607,10.);
#5322=VECTOR('',#18608,10.);
#5323=VECTOR('',#18609,10.);
#5324=VECTOR('',#18610,10.);
#5325=VECTOR('',#18611,10.);
#5326=VECTOR('',#18612,10.);
#5327=VECTOR('',#18613,10.);
#5328=VECTOR('',#18614,10.);
#5329=VECTOR('',#18619,10.);
#5330=VECTOR('',#18620,10.);
#5331=VECTOR('',#18621,10.);
#5332=VECTOR('',#18624,10.);
#5333=VECTOR('',#18625,10.);
#5334=VECTOR('',#18628,10.);
#5335=VECTOR('',#18629,10.);
#5336=VECTOR('',#18632,10.);
#5337=VECTOR('',#18633,10.);
#5338=VECTOR('',#18636,10.);
#5339=VECTOR('',#18637,10.);
#5340=VECTOR('',#18640,10.);
#5341=VECTOR('',#18641,10.);
#5342=VECTOR('',#18644,10.);
#5343=VECTOR('',#18645,10.);
#5344=VECTOR('',#18648,10.);
#5345=VECTOR('',#18651,10.);
#5346=VECTOR('',#18652,10.);
#5347=VECTOR('',#18653,10.);
#5348=VECTOR('',#18654,10.);
#5349=VECTOR('',#18655,10.);
#5350=VECTOR('',#18656,10.);
#5351=VECTOR('',#18657,10.);
#5352=VECTOR('',#18658,10.);
#5353=VECTOR('',#18659,10.);
#5354=VECTOR('',#18660,10.);
#5355=VECTOR('',#18661,10.);
#5356=VECTOR('',#18662,10.);
#5357=VECTOR('',#18663,10.);
#5358=VECTOR('',#18664,10.);
#5359=VECTOR('',#18665,10.);
#5360=VECTOR('',#18666,10.);
#5361=VECTOR('',#18671,10.);
#5362=VECTOR('',#18672,10.);
#5363=VECTOR('',#18673,10.);
#5364=VECTOR('',#18676,10.);
#5365=VECTOR('',#18677,10.);
#5366=VECTOR('',#18680,10.);
#5367=VECTOR('',#18681,10.);
#5368=VECTOR('',#18684,10.);
#5369=VECTOR('',#18685,10.);
#5370=VECTOR('',#18688,10.);
#5371=VECTOR('',#18689,10.);
#5372=VECTOR('',#18692,10.);
#5373=VECTOR('',#18693,10.);
#5374=VECTOR('',#18696,10.);
#5375=VECTOR('',#18697,10.);
#5376=VECTOR('',#18700,10.);
#5377=VECTOR('',#18701,10.);
#5378=VECTOR('',#18704,10.);
#5379=VECTOR('',#18705,10.);
#5380=VECTOR('',#18708,10.);
#5381=VECTOR('',#18713,3.05);
#5382=VECTOR('',#18722,21.525);
#5383=VECTOR('',#18725,21.05);
#6508=CIRCLE('',#16761,15.2);
#6509=CIRCLE('',#16762,15.2);
#6510=CIRCLE('',#16763,15.7);
#6511=CIRCLE('',#16765,15.2);
#6512=CIRCLE('',#16767,21.05);
#6513=CIRCLE('',#16769,15.7);
#6514=CIRCLE('',#16771,25.5);
#6515=CIRCLE('',#16772,25.5);
#6516=CIRCLE('',#16773,25.5);
#6517=CIRCLE('',#16777,4.5);
#6518=CIRCLE('',#16778,4.5);
#6519=CIRCLE('',#16780,1.5);
#6520=CIRCLE('',#16785,1.5);
#6521=CIRCLE('',#16788,1.5);
#6522=CIRCLE('',#16791,1.5);
#6523=CIRCLE('',#16792,1.5);
#6524=CIRCLE('',#16794,1.5);
#6525=CIRCLE('',#16795,1.5);
#6526=CIRCLE('',#16797,1.5);
#6527=CIRCLE('',#16798,1.5);
#6528=CIRCLE('',#16803,1.5);
#6529=CIRCLE('',#16804,1.5);
#6530=CIRCLE('',#16805,1.5);
#6531=CIRCLE('',#16809,1.5);
#6532=CIRCLE('',#16810,1.5);
#6533=CIRCLE('',#16811,1.5);
#6534=CIRCLE('',#16813,1.49999999999999);
#6535=CIRCLE('',#16814,1.5);
#6536=CIRCLE('',#16818,1.50000000000001);
#6537=CIRCLE('',#16819,1.5);
#6538=CIRCLE('',#16820,1.5);
#6539=CIRCLE('',#16822,1.49999999999999);
#6540=CIRCLE('',#16823,1.5);
#6541=CIRCLE('',#16824,1.5);
#6542=CIRCLE('',#16828,1.5);
#6543=CIRCLE('',#16829,1.5);
#6544=CIRCLE('',#16831,1.5);
#6545=CIRCLE('',#16832,1.5);
#6546=CIRCLE('',#16833,1.5);
#6547=CIRCLE('',#16837,1.5);
#6548=CIRCLE('',#16838,1.5);
#6549=CIRCLE('',#16839,1.5);
#6550=CIRCLE('',#16841,1.5);
#6551=CIRCLE('',#16843,1.5);
#6552=CIRCLE('',#16844,1.5);
#6553=CIRCLE('',#16846,1.5);
#6554=CIRCLE('',#16849,1.5);
#6555=CIRCLE('',#16850,1.5);
#6556=CIRCLE('',#16851,1.5);
#6557=CIRCLE('',#16854,1.5);
#6558=CIRCLE('',#16860,1.5);
#6559=CIRCLE('',#16864,1.5);
#6560=CIRCLE('',#16868,27.);
#6561=CIRCLE('',#16870,27.);
#6562=CIRCLE('',#16875,1.5);
#6563=CIRCLE('',#16876,1.5);
#6564=CIRCLE('',#16877,1.5);
#6565=CIRCLE('',#16881,1.5);
#6566=CIRCLE('',#16882,1.5);
#6567=CIRCLE('',#16883,1.5);
#6568=CIRCLE('',#16889,27.);
#6569=CIRCLE('',#16891,25.3786796564404);
#6570=CIRCLE('',#16892,1.5);
#6571=CIRCLE('',#16893,26.4393398282202);
#6572=CIRCLE('',#16894,26.4393398282202);
#6573=CIRCLE('',#16896,26.5606601717798);
#6574=CIRCLE('',#16897,26.5606601717798);
#6575=CIRCLE('',#16899,21.905);
#6576=CIRCLE('',#16901,1.5);
#6577=CIRCLE('',#16902,27.);
#6578=CIRCLE('',#16903,27.);
#6579=CIRCLE('',#16905,27.);
#6580=CIRCLE('',#16906,27.);
#6581=CIRCLE('',#16907,27.);
#6582=CIRCLE('',#16908,27.);
#6583=CIRCLE('',#16909,27.);
#6584=CIRCLE('',#16912,1.5);
#6585=CIRCLE('',#16913,1.5);
#6586=CIRCLE('',#16915,4.5);
#6587=CIRCLE('',#16916,3.);
#6588=CIRCLE('',#16918,1.5);
#6589=CIRCLE('',#16919,1.5);
#6590=CIRCLE('',#16921,1.5);
#6591=CIRCLE('',#16922,3.);
#6592=CIRCLE('',#16925,3.);
#6593=CIRCLE('',#16928,1.5);
#6594=CIRCLE('',#16929,3.);
#6595=CIRCLE('',#16930,4.5);
#6596=CIRCLE('',#16934,3.05);
#6597=CIRCLE('',#16961,3.05);
#6598=CIRCLE('',#16964,21.05);
#6963=VERTEX_POINT('',#22167);
#6964=VERTEX_POINT('',#22168);
#6965=VERTEX_POINT('',#22171);
#6966=VERTEX_POINT('',#22175);
#6967=VERTEX_POINT('',#22179);
#6968=VERTEX_POINT('',#22182);
#6969=VERTEX_POINT('',#22186);
#6970=VERTEX_POINT('',#22187);
#6971=VERTEX_POINT('',#22189);
#6972=VERTEX_POINT('',#22191);
#6973=VERTEX_POINT('',#22193);
#6974=VERTEX_POINT('',#22195);
#6975=VERTEX_POINT('',#22197);
#6976=VERTEX_POINT('',#22199);
#6977=VERTEX_POINT('',#22201);
#6978=VERTEX_POINT('',#22203);
#6979=VERTEX_POINT('',#22230);
#6980=VERTEX_POINT('',#22231);
#6981=VERTEX_POINT('',#22287);
#6982=VERTEX_POINT('',#22292);
#6983=VERTEX_POINT('',#22369);
#6984=VERTEX_POINT('',#22375);
#6985=VERTEX_POINT('',#22383);
#6986=VERTEX_POINT('',#22384);
#6987=VERTEX_POINT('',#22389);
#6988=VERTEX_POINT('',#22391);
#6989=VERTEX_POINT('',#22393);
#6990=VERTEX_POINT('',#22395);
#6991=VERTEX_POINT('',#22397);
#6992=VERTEX_POINT('',#22399);
#6993=VERTEX_POINT('',#22401);
#6994=VERTEX_POINT('',#22403);
#6995=VERTEX_POINT('',#22405);
#6996=VERTEX_POINT('',#22407);
#6997=VERTEX_POINT('',#22409);
#6998=VERTEX_POINT('',#22411);
#6999=VERTEX_POINT('',#22415);
#7000=VERTEX_POINT('',#22419);
#7001=VERTEX_POINT('',#22421);
#7002=VERTEX_POINT('',#22423);
#7003=VERTEX_POINT('',#22450);
#7004=VERTEX_POINT('',#22451);
#7005=VERTEX_POINT('',#22507);
#7006=VERTEX_POINT('',#22512);
#7007=VERTEX_POINT('',#22593);
#7008=VERTEX_POINT('',#22594);
#7009=VERTEX_POINT('',#22650);
#7010=VERTEX_POINT('',#22655);
#7011=VERTEX_POINT('',#22728);
#7012=VERTEX_POINT('',#22733);
#7013=VERTEX_POINT('',#22755);
#7014=VERTEX_POINT('',#22756);
#7015=VERTEX_POINT('',#22758);
#7016=VERTEX_POINT('',#22763);
#7017=VERTEX_POINT('',#22794);
#7018=VERTEX_POINT('',#22795);
#7019=VERTEX_POINT('',#22797);
#7020=VERTEX_POINT('',#22799);
#7021=VERTEX_POINT('',#22842);
#7022=VERTEX_POINT('',#22843);
#7023=VERTEX_POINT('',#22845);
#7024=VERTEX_POINT('',#22850);
#7025=VERTEX_POINT('',#22896);
#7026=VERTEX_POINT('',#22901);
#7027=VERTEX_POINT('',#22932);
#7028=VERTEX_POINT('',#22934);
#7029=VERTEX_POINT('',#22938);
#7030=VERTEX_POINT('',#22940);
#7031=VERTEX_POINT('',#22944);
#7032=VERTEX_POINT('',#22948);
#7033=VERTEX_POINT('',#22952);
#7034=VERTEX_POINT('',#22953);
#7035=VERTEX_POINT('',#22955);
#7036=VERTEX_POINT('',#22957);
#7037=VERTEX_POINT('',#22961);
#7038=VERTEX_POINT('',#22968);
#7039=VERTEX_POINT('',#22970);
#7040=VERTEX_POINT('',#22985);
#7041=VERTEX_POINT('',#22987);
#7042=VERTEX_POINT('',#23000);
#7043=VERTEX_POINT('',#23004);
#7044=VERTEX_POINT('',#23006);
#7045=VERTEX_POINT('',#23010);
#7046=VERTEX_POINT('',#23021);
#7047=VERTEX_POINT('',#23022);
#7048=VERTEX_POINT('',#23038);
#7049=VERTEX_POINT('',#23039);
#7050=VERTEX_POINT('',#23044);
#7051=VERTEX_POINT('',#23052);
#7052=VERTEX_POINT('',#23053);
#7053=VERTEX_POINT('',#23055);
#7054=VERTEX_POINT('',#23059);
#7055=VERTEX_POINT('',#23060);
#7056=VERTEX_POINT('',#23071);
#7057=VERTEX_POINT('',#23075);
#7058=VERTEX_POINT('',#23085);
#7059=VERTEX_POINT('',#23090);
#7060=VERTEX_POINT('',#23094);
#7061=VERTEX_POINT('',#23102);
#7062=VERTEX_POINT('',#23103);
#7063=VERTEX_POINT('',#23105);
#7064=VERTEX_POINT('',#23115);
#7065=VERTEX_POINT('',#23116);
#7066=VERTEX_POINT('',#23120);
#7067=VERTEX_POINT('',#23124);
#7068=VERTEX_POINT('',#23128);
#7069=VERTEX_POINT('',#23132);
#7070=VERTEX_POINT('',#23136);
#7071=VERTEX_POINT('',#23140);
#7072=VERTEX_POINT('',#23144);
#7073=VERTEX_POINT('',#23148);
#7074=VERTEX_POINT('',#23152);
#7075=VERTEX_POINT('',#23159);
#7076=VERTEX_POINT('',#23160);
#7077=VERTEX_POINT('',#23162);
#7078=VERTEX_POINT('',#23164);
#7079=VERTEX_POINT('',#23166);
#7080=VERTEX_POINT('',#23168);
#7081=VERTEX_POINT('',#23170);
#7082=VERTEX_POINT('',#23172);
#7083=VERTEX_POINT('',#23175);
#7084=VERTEX_POINT('',#23176);
#7085=VERTEX_POINT('',#23180);
#7086=VERTEX_POINT('',#23184);
#7087=VERTEX_POINT('',#23188);
#7088=VERTEX_POINT('',#23192);
#7089=VERTEX_POINT('',#23196);
#7090=VERTEX_POINT('',#23200);
#7091=VERTEX_POINT('',#23204);
#7092=VERTEX_POINT('',#23208);
#7093=VERTEX_POINT('',#23212);
#7094=VERTEX_POINT('',#23216);
#7095=VERTEX_POINT('',#23220);
#7096=VERTEX_POINT('',#23224);
#7097=VERTEX_POINT('',#23228);
#7098=VERTEX_POINT('',#23232);
#7099=VERTEX_POINT('',#23239);
#7100=VERTEX_POINT('',#23240);
#7101=VERTEX_POINT('',#23242);
#7102=VERTEX_POINT('',#23244);
#7103=VERTEX_POINT('',#23246);
#7104=VERTEX_POINT('',#23248);
#7105=VERTEX_POINT('',#23250);
#7106=VERTEX_POINT('',#23252);
#7107=VERTEX_POINT('',#23254);
#7108=VERTEX_POINT('',#23256);
#7109=VERTEX_POINT('',#23264);
#7110=VERTEX_POINT('',#23272);
#7111=VERTEX_POINT('',#23274);
#7112=VERTEX_POINT('',#23279);
#7113=VERTEX_POINT('',#23298);
#7114=VERTEX_POINT('',#23332);
#7115=VERTEX_POINT('',#23333);
#7116=VERTEX_POINT('',#23338);
#7117=VERTEX_POINT('',#23355);
#7118=VERTEX_POINT('',#23372);
#7119=VERTEX_POINT('',#23373);
#7120=VERTEX_POINT('',#23375);
#7121=VERTEX_POINT('',#23382);
#7122=VERTEX_POINT('',#23386);
#7123=VERTEX_POINT('',#23399);
#7124=VERTEX_POINT('',#23401);
#7125=VERTEX_POINT('',#23418);
#7126=VERTEX_POINT('',#23420);
#7127=VERTEX_POINT('',#23422);
#7128=VERTEX_POINT('',#23426);
#7129=VERTEX_POINT('',#23428);
#7130=VERTEX_POINT('',#23432);
#7131=VERTEX_POINT('',#23435);
#7132=VERTEX_POINT('',#23437);
#7133=VERTEX_POINT('',#23441);
#7134=VERTEX_POINT('',#23446);
#7135=VERTEX_POINT('',#23453);
#7136=VERTEX_POINT('',#23454);
#7137=VERTEX_POINT('',#23456);
#7138=VERTEX_POINT('',#23458);
#7139=VERTEX_POINT('',#23465);
#7140=VERTEX_POINT('',#23467);
#7141=VERTEX_POINT('',#23492);
#7142=VERTEX_POINT('',#23515);
#7143=VERTEX_POINT('',#23528);
#7144=VERTEX_POINT('',#23530);
#7145=VERTEX_POINT('',#23541);
#7146=VERTEX_POINT('',#23552);
#7147=VERTEX_POINT('',#23563);
#7148=VERTEX_POINT('',#23574);
#7149=VERTEX_POINT('',#23585);
#7150=VERTEX_POINT('',#23596);
#7151=VERTEX_POINT('',#23607);
#7152=VERTEX_POINT('',#23618);
#7153=VERTEX_POINT('',#23629);
#7154=VERTEX_POINT('',#23645);
#7155=VERTEX_POINT('',#23647);
#7156=VERTEX_POINT('',#23651);
#7157=VERTEX_POINT('',#23655);
#7158=VERTEX_POINT('',#23659);
#7159=VERTEX_POINT('',#23663);
#7160=VERTEX_POINT('',#23667);
#7161=VERTEX_POINT('',#23671);
#7162=VERTEX_POINT('',#23683);
#7163=VERTEX_POINT('',#23685);
#7164=VERTEX_POINT('',#23696);
#7165=VERTEX_POINT('',#23707);
#7166=VERTEX_POINT('',#23718);
#7167=VERTEX_POINT('',#23729);
#7168=VERTEX_POINT('',#23740);
#7169=VERTEX_POINT('',#23751);
#7170=VERTEX_POINT('',#23762);
#7171=VERTEX_POINT('',#23773);
#7172=VERTEX_POINT('',#23784);
#7173=VERTEX_POINT('',#23795);
#7174=VERTEX_POINT('',#23806);
#7175=VERTEX_POINT('',#23817);
#7176=VERTEX_POINT('',#23828);
#7177=VERTEX_POINT('',#23839);
#7178=VERTEX_POINT('',#23855);
#7179=VERTEX_POINT('',#23857);
#7180=VERTEX_POINT('',#23861);
#7181=VERTEX_POINT('',#23865);
#7182=VERTEX_POINT('',#23869);
#7183=VERTEX_POINT('',#23873);
#7184=VERTEX_POINT('',#23877);
#7185=VERTEX_POINT('',#23881);
#7186=VERTEX_POINT('',#23885);
#7187=VERTEX_POINT('',#23889);
#7188=VERTEX_POINT('',#23896);
#7189=VERTEX_POINT('',#23901);
#8464=EDGE_CURVE('',#6963,#6964,#6508,.T.);
#8465=EDGE_CURVE('',#6964,#6963,#6509,.T.);
#8466=EDGE_CURVE('',#6963,#6965,#3886,.T.);
#8467=EDGE_CURVE('',#6965,#6965,#6510,.T.);
#8468=EDGE_CURVE('',#6966,#6966,#6511,.T.);
#8469=EDGE_CURVE('',#6966,#6964,#3887,.T.);
#8470=EDGE_CURVE('',#6967,#6967,#6512,.T.);
#8471=EDGE_CURVE('',#6968,#6968,#6513,.T.);
#8472=EDGE_CURVE('',#6968,#6966,#3888,.T.);
#8473=EDGE_CURVE('',#6969,#6970,#6514,.T.);
#8474=EDGE_CURVE('',#6971,#6969,#3889,.T.);
#8475=EDGE_CURVE('',#6972,#6971,#3890,.T.);
#8476=EDGE_CURVE('',#6973,#6972,#3891,.T.);
#8477=EDGE_CURVE('',#6974,#6973,#6515,.T.);
#8478=EDGE_CURVE('',#6975,#6974,#3892,.T.);
#8479=EDGE_CURVE('',#6976,#6975,#3893,.T.);
#8480=EDGE_CURVE('',#6977,#6976,#6516,.T.);
#8481=EDGE_CURVE('',#6978,#6977,#3894,.T.);
#8482=EDGE_CURVE('',#6970,#6978,#3895,.T.);
#8483=EDGE_CURVE('',#6979,#6980,#256,.T.);
#8484=EDGE_CURVE('',#6981,#6980,#257,.T.);
#8485=EDGE_CURVE('',#6981,#6982,#258,.T.);
#8486=EDGE_CURVE('',#6982,#6979,#3896,.T.);
#8487=EDGE_CURVE('',#6980,#6983,#259,.T.);
#8488=EDGE_CURVE('',#6983,#6984,#3897,.T.);
#8489=EDGE_CURVE('',#6984,#6981,#260,.T.);
#8490=EDGE_CURVE('',#6985,#6986,#246,.F.);
#8491=EDGE_CURVE('',#6986,#6984,#3898,.T.);
#8492=EDGE_CURVE('',#6983,#6985,#3899,.T.);
#8493=EDGE_CURVE('',#6987,#6982,#3900,.T.);
#8494=EDGE_CURVE('',#6988,#6987,#3901,.T.);
#8495=EDGE_CURVE('',#6989,#6988,#3902,.T.);
#8496=EDGE_CURVE('',#6990,#6989,#3903,.T.);
#8497=EDGE_CURVE('',#6991,#6990,#3904,.T.);
#8498=EDGE_CURVE('',#6992,#6991,#3905,.T.);
#8499=EDGE_CURVE('',#6993,#6992,#3906,.T.);
#8500=EDGE_CURVE('',#6994,#6993,#6517,.T.);
#8501=EDGE_CURVE('',#6995,#6994,#3907,.T.);
#8502=EDGE_CURVE('',#6996,#6995,#6518,.T.);
#8503=EDGE_CURVE('',#6997,#6996,#3908,.T.);
#8504=EDGE_CURVE('',#6997,#6998,#3909,.T.);
#8505=EDGE_CURVE('',#6979,#6998,#3910,.T.);
#8506=EDGE_CURVE('',#6984,#6999,#3911,.T.);
#8507=EDGE_CURVE('',#6987,#6999,#6519,.T.);
#8508=EDGE_CURVE('',#6986,#7000,#247,.T.);
#8509=EDGE_CURVE('',#7001,#7000,#3912,.T.);
#8510=EDGE_CURVE('',#7002,#7001,#3913,.T.);
#8511=EDGE_CURVE('',#6999,#7002,#3914,.T.);
#8512=EDGE_CURVE('',#7003,#7004,#261,.T.);
#8513=EDGE_CURVE('',#7005,#7004,#262,.T.);
#8514=EDGE_CURVE('',#7005,#7006,#263,.T.);
#8515=EDGE_CURVE('',#7006,#7003,#3915,.T.);
#8516=EDGE_CURVE('',#7007,#7008,#264,.T.);
#8517=EDGE_CURVE('',#7009,#7008,#265,.T.);
#8518=EDGE_CURVE('',#7009,#7010,#266,.T.);
#8519=EDGE_CURVE('',#7010,#7007,#3916,.T.);
#8520=EDGE_CURVE('',#7008,#7011,#267,.T.);
#8521=EDGE_CURVE('',#7011,#7012,#3917,.T.);
#8522=EDGE_CURVE('',#7012,#7009,#268,.T.);
#8523=EDGE_CURVE('',#7013,#7014,#3918,.T.);
#8524=EDGE_CURVE('',#7014,#7015,#269,.T.);
#8525=EDGE_CURVE('',#7015,#7016,#3919,.T.);
#8526=EDGE_CURVE('',#7016,#7013,#270,.T.);
#8527=EDGE_CURVE('',#7015,#7012,#271,.T.);
#8528=EDGE_CURVE('',#7011,#7016,#272,.T.);
#8529=EDGE_CURVE('',#7017,#7018,#3920,.T.);
#8530=EDGE_CURVE('',#7018,#7019,#3921,.T.);
#8531=EDGE_CURVE('',#7019,#7020,#3922,.T.);
#8532=EDGE_CURVE('',#7020,#7017,#3923,.T.);
#8533=EDGE_CURVE('',#7017,#7014,#273,.T.);
#8534=EDGE_CURVE('',#7013,#7018,#274,.T.);
#8535=EDGE_CURVE('',#7021,#7022,#3924,.T.);
#8536=EDGE_CURVE('',#7022,#7023,#275,.T.);
#8537=EDGE_CURVE('',#7023,#7024,#3925,.T.);
#8538=EDGE_CURVE('',#7024,#7021,#276,.T.);
#8539=EDGE_CURVE('',#7021,#7020,#277,.T.);
#8540=EDGE_CURVE('',#7019,#7022,#278,.T.);
#8541=EDGE_CURVE('',#7004,#7025,#279,.T.);
#8542=EDGE_CURVE('',#7025,#7026,#3926,.T.);
#8543=EDGE_CURVE('',#7026,#7005,#280,.T.);
#8544=EDGE_CURVE('',#7025,#7024,#281,.T.);
#8545=EDGE_CURVE('',#7023,#7026,#282,.T.);
#8546=EDGE_CURVE('',#7007,#7027,#3927,.T.);
#8547=EDGE_CURVE('',#7027,#7028,#6520,.F.);
#8548=EDGE_CURVE('',#7028,#7013,#3928,.T.);
#8549=EDGE_CURVE('',#7029,#7010,#3929,.T.);
#8550=EDGE_CURVE('',#7030,#7029,#3930,.T.);
#8551=EDGE_CURVE('',#7027,#7030,#3931,.T.);
#8552=EDGE_CURVE('',#7012,#7031,#3932,.T.);
#8553=EDGE_CURVE('',#7031,#7029,#6521,.T.);
#8554=EDGE_CURVE('',#7032,#7025,#3933,.T.);
#8555=EDGE_CURVE('',#7031,#7032,#3934,.T.);
#8556=EDGE_CURVE('',#7033,#7034,#6522,.T.);
#8557=EDGE_CURVE('',#7034,#7035,#3935,.T.);
#8558=EDGE_CURVE('',#7035,#7036,#6523,.T.);
#8559=EDGE_CURVE('',#7036,#7033,#3936,.T.);
#8560=EDGE_CURVE('',#7035,#7037,#6524,.T.);
#8561=EDGE_CURVE('',#7037,#7036,#6525,.T.);
#8562=EDGE_CURVE('',#7033,#6978,#6526,.T.);
#8563=EDGE_CURVE('',#6978,#7034,#6527,.T.);
#8564=EDGE_CURVE('',#7037,#7038,#3937,.T.);
#8565=EDGE_CURVE('',#7038,#7039,#283,.F.);
#8566=EDGE_CURVE('',#7039,#7036,#3938,.T.);
#8567=EDGE_CURVE('',#7035,#7040,#3939,.T.);
#8568=EDGE_CURVE('',#7040,#7041,#284,.F.);
#8569=EDGE_CURVE('',#7041,#7037,#3940,.T.);
#8570=EDGE_CURVE('',#7042,#7034,#3941,.T.);
#8571=EDGE_CURVE('',#7042,#7040,#3942,.T.);
#8572=EDGE_CURVE('',#7001,#7043,#6528,.F.);
#8573=EDGE_CURVE('',#7044,#7001,#6529,.F.);
#8574=EDGE_CURVE('',#7043,#7044,#6530,.F.);
#8575=EDGE_CURVE('',#7000,#7045,#285,.F.);
#8576=EDGE_CURVE('',#7045,#7044,#3943,.T.);
#8577=EDGE_CURVE('',#7046,#7047,#286,.F.);
#8578=EDGE_CURVE('',#7047,#7043,#3944,.T.);
#8579=EDGE_CURVE('',#7044,#7046,#3945,.T.);
#8580=EDGE_CURVE('',#7048,#7049,#6531,.F.);
#8581=EDGE_CURVE('',#7002,#7048,#6532,.F.);
#8582=EDGE_CURVE('',#7049,#7002,#6533,.F.);
#8583=EDGE_CURVE('',#6999,#7050,#6534,.T.);
#8584=EDGE_CURVE('',#7050,#6987,#6535,.T.);
#8585=EDGE_CURVE('',#7048,#7050,#3946,.T.);
#8586=EDGE_CURVE('',#7043,#7049,#3947,.T.);
#8587=EDGE_CURVE('',#7051,#7052,#6536,.F.);
#8588=EDGE_CURVE('',#7053,#7051,#6537,.F.);
#8589=EDGE_CURVE('',#7052,#7053,#6538,.F.);
#8590=EDGE_CURVE('',#7054,#7055,#6539,.T.);
#8591=EDGE_CURVE('',#7055,#6988,#6540,.T.);
#8592=EDGE_CURVE('',#6988,#7054,#6541,.T.);
#8593=EDGE_CURVE('',#7054,#7053,#3948,.T.);
#8594=EDGE_CURVE('',#7051,#7055,#3949,.T.);
#8595=EDGE_CURVE('',#7049,#7052,#3950,.T.);
#8596=EDGE_CURVE('',#7053,#7048,#3951,.T.);
#8597=EDGE_CURVE('',#7056,#7027,#6542,.F.);
#8598=EDGE_CURVE('',#7028,#7056,#6543,.F.);
#8599=EDGE_CURVE('',#7057,#7030,#6544,.T.);
#8600=EDGE_CURVE('',#7030,#6989,#6545,.T.);
#8601=EDGE_CURVE('',#6989,#7057,#6546,.T.);
#8602=EDGE_CURVE('',#7057,#7056,#3952,.T.);
#8603=EDGE_CURVE('',#7052,#7028,#3953,.T.);
#8604=EDGE_CURVE('',#7056,#7051,#3954,.T.);
#8605=EDGE_CURVE('',#7058,#7032,#6547,.F.);
#8606=EDGE_CURVE('',#6991,#7058,#6548,.F.);
#8607=EDGE_CURVE('',#7032,#6991,#6549,.F.);
#8608=EDGE_CURVE('',#7059,#6992,#6550,.T.);
#8609=EDGE_CURVE('',#7058,#7059,#3955,.T.);
#8610=EDGE_CURVE('',#7059,#7060,#6551,.T.);
#8611=EDGE_CURVE('',#7060,#6992,#6552,.T.);
#8612=EDGE_CURVE('',#6990,#7031,#6553,.T.);
#8613=EDGE_CURVE('',#7003,#7058,#3956,.T.);
#8614=EDGE_CURVE('',#7061,#7062,#6554,.T.);
#8615=EDGE_CURVE('',#7062,#7063,#6555,.T.);
#8616=EDGE_CURVE('',#7063,#7061,#6556,.T.);
#8617=EDGE_CURVE('',#7022,#7062,#3957,.T.);
#8618=EDGE_CURVE('',#7061,#7006,#3958,.T.);
#8619=EDGE_CURVE('',#6990,#7029,#6557,.T.);
#8620=EDGE_CURVE('',#7050,#7054,#3959,.T.);
#8621=EDGE_CURVE('',#7064,#7065,#287,.T.);
#8622=EDGE_CURVE('',#7065,#7066,#288,.T.);
#8623=EDGE_CURVE('',#7066,#7067,#289,.T.);
#8624=EDGE_CURVE('',#7067,#7068,#290,.T.);
#8625=EDGE_CURVE('',#7068,#7069,#291,.T.);
#8626=EDGE_CURVE('',#7069,#7070,#292,.T.);
#8627=EDGE_CURVE('',#7070,#7071,#293,.T.);
#8628=EDGE_CURVE('',#7071,#7072,#294,.T.);
#8629=EDGE_CURVE('',#7072,#7073,#295,.T.);
#8630=EDGE_CURVE('',#7073,#7074,#296,.T.);
#8631=EDGE_CURVE('',#7074,#7064,#297,.T.);
#8632=EDGE_CURVE('',#7075,#7076,#3960,.T.);
#8633=EDGE_CURVE('',#7076,#7077,#3961,.T.);
#8634=EDGE_CURVE('',#7077,#7078,#3962,.T.);
#8635=EDGE_CURVE('',#7078,#7079,#3963,.T.);
#8636=EDGE_CURVE('',#7079,#7080,#3964,.T.);
#8637=EDGE_CURVE('',#7080,#7081,#3965,.T.);
#8638=EDGE_CURVE('',#7081,#7082,#3966,.T.);
#8639=EDGE_CURVE('',#7082,#7075,#3967,.T.);
#8640=EDGE_CURVE('',#7083,#7084,#298,.T.);
#8641=EDGE_CURVE('',#7084,#7085,#299,.T.);
#8642=EDGE_CURVE('',#7085,#7086,#300,.T.);
#8643=EDGE_CURVE('',#7086,#7087,#301,.T.);
#8644=EDGE_CURVE('',#7087,#7088,#302,.T.);
#8645=EDGE_CURVE('',#7088,#7089,#303,.T.);
#8646=EDGE_CURVE('',#7089,#7090,#304,.T.);
#8647=EDGE_CURVE('',#7090,#7091,#305,.T.);
#8648=EDGE_CURVE('',#7091,#7092,#306,.T.);
#8649=EDGE_CURVE('',#7092,#7093,#307,.T.);
#8650=EDGE_CURVE('',#7093,#7094,#308,.T.);
#8651=EDGE_CURVE('',#7094,#7095,#309,.T.);
#8652=EDGE_CURVE('',#7095,#7096,#310,.T.);
#8653=EDGE_CURVE('',#7096,#7097,#311,.T.);
#8654=EDGE_CURVE('',#7097,#7098,#312,.T.);
#8655=EDGE_CURVE('',#7098,#7083,#313,.T.);
#8656=EDGE_CURVE('',#7099,#7100,#3968,.T.);
#8657=EDGE_CURVE('',#7100,#7101,#3969,.T.);
#8658=EDGE_CURVE('',#7101,#7102,#3970,.T.);
#8659=EDGE_CURVE('',#7102,#7103,#3971,.T.);
#8660=EDGE_CURVE('',#7103,#7104,#3972,.T.);
#8661=EDGE_CURVE('',#7104,#7105,#3973,.T.);
#8662=EDGE_CURVE('',#7105,#7106,#3974,.T.);
#8663=EDGE_CURVE('',#7106,#7107,#3975,.T.);
#8664=EDGE_CURVE('',#7107,#7108,#3976,.T.);
#8665=EDGE_CURVE('',#7108,#7099,#3977,.T.);
#8666=EDGE_CURVE('',#7055,#7057,#3978,.T.);
#8667=EDGE_CURVE('',#7060,#7109,#3979,.T.);
#8668=EDGE_CURVE('',#6993,#7109,#6558,.T.);
#8669=EDGE_CURVE('',#7059,#7061,#3980,.T.);
#8670=EDGE_CURVE('',#7063,#7060,#3981,.T.);
#8671=EDGE_CURVE('',#7062,#7110,#3982,.T.);
#8672=EDGE_CURVE('',#7111,#7110,#6559,.T.);
#8673=EDGE_CURVE('',#7111,#7063,#3983,.T.);
#8674=EDGE_CURVE('',#6998,#7112,#314,.F.);
#8675=EDGE_CURVE('',#7112,#6983,#3984,.T.);
#8676=EDGE_CURVE('',#7112,#6985,#6560,.T.);
#8677=EDGE_CURVE('',#7041,#7038,#6561,.T.);
#8678=EDGE_CURVE('',#7033,#7113,#3985,.T.);
#8679=EDGE_CURVE('',#7113,#6970,#315,.F.);
#8680=EDGE_CURVE('',#6977,#7042,#316,.F.);
#8681=EDGE_CURVE('',#7039,#7113,#3986,.T.);
#8682=EDGE_CURVE('',#7114,#7115,#6562,.F.);
#8683=EDGE_CURVE('',#6975,#7114,#6563,.F.);
#8684=EDGE_CURVE('',#7115,#6975,#6564,.F.);
#8685=EDGE_CURVE('',#7116,#6976,#317,.F.);
#8686=EDGE_CURVE('',#7114,#7116,#3987,.T.);
#8687=EDGE_CURVE('',#6974,#7117,#318,.F.);
#8688=EDGE_CURVE('',#7117,#7115,#3988,.T.);
#8689=EDGE_CURVE('',#7118,#7119,#6565,.T.);
#8690=EDGE_CURVE('',#7119,#7120,#6566,.T.);
#8691=EDGE_CURVE('',#7120,#7118,#6567,.T.);
#8692=EDGE_CURVE('',#7118,#7114,#3989,.T.);
#8693=EDGE_CURVE('',#7115,#7119,#3990,.T.);
#8694=EDGE_CURVE('',#7121,#7118,#3991,.T.);
#8695=EDGE_CURVE('',#7121,#7116,#3992,.T.);
#8696=EDGE_CURVE('',#7120,#7122,#3993,.T.);
#8697=EDGE_CURVE('',#7122,#7121,#319,.F.);
#8698=EDGE_CURVE('',#7119,#7123,#3994,.T.);
#8699=EDGE_CURVE('',#7123,#7124,#320,.F.);
#8700=EDGE_CURVE('',#7124,#7120,#3995,.T.);
#8701=EDGE_CURVE('',#7124,#7122,#6568,.T.);
#8702=EDGE_CURVE('',#7125,#7125,#6569,.T.);
#8703=EDGE_CURVE('',#7125,#7126,#6570,.T.);
#8704=EDGE_CURVE('',#7126,#7127,#6571,.T.);
#8705=EDGE_CURVE('',#7127,#7126,#6572,.T.);
#8706=EDGE_CURVE('',#7127,#7128,#3996,.T.);
#8707=EDGE_CURVE('',#7129,#7128,#6573,.T.);
#8708=EDGE_CURVE('',#7128,#7129,#6574,.T.);
#8709=EDGE_CURVE('',#7130,#7130,#6575,.T.);
#8710=EDGE_CURVE('',#7129,#7131,#6576,.T.);
#8711=EDGE_CURVE('',#7131,#7132,#6577,.T.);
#8712=EDGE_CURVE('',#7132,#7131,#6578,.T.);
#8713=EDGE_CURVE('',#7132,#7133,#3997,.T.);
#8714=EDGE_CURVE('',#7113,#7133,#6579,.T.);
#8715=EDGE_CURVE('',#7116,#7042,#6580,.T.);
#8716=EDGE_CURVE('',#7117,#7123,#3998,.T.);
#8717=EDGE_CURVE('',#7134,#7117,#6581,.T.);
#8718=EDGE_CURVE('',#7047,#7134,#3999,.T.);
#8719=EDGE_CURVE('',#7045,#7046,#6582,.T.);
#8720=EDGE_CURVE('',#7133,#6997,#6583,.T.);
#8721=EDGE_CURVE('',#7135,#7136,#6584,.T.);
#8722=EDGE_CURVE('',#7136,#7137,#4000,.T.);
#8723=EDGE_CURVE('',#7137,#7138,#6585,.T.);
#8724=EDGE_CURVE('',#7138,#7135,#4001,.T.);
#8725=EDGE_CURVE('',#7110,#7138,#6586,.T.);
#8726=EDGE_CURVE('',#7137,#7111,#6587,.T.);
#8727=EDGE_CURVE('',#6994,#7139,#6588,.T.);
#8728=EDGE_CURVE('',#7139,#7140,#4002,.T.);
#8729=EDGE_CURVE('',#7140,#6995,#6589,.T.);
#8730=EDGE_CURVE('',#6971,#6996,#6590,.T.);
#8731=EDGE_CURVE('',#7140,#6971,#6591,.T.);
#8732=EDGE_CURVE('',#6969,#6997,#321,.T.);
#8733=EDGE_CURVE('',#7109,#7139,#6592,.T.);
#8734=EDGE_CURVE('',#7141,#6972,#6593,.T.);
#8735=EDGE_CURVE('',#6972,#7136,#6594,.T.);
#8736=EDGE_CURVE('',#7135,#7141,#6595,.T.);
#8737=EDGE_CURVE('',#7141,#7134,#4003,.T.);
#8738=EDGE_CURVE('',#7134,#6973,#322,.T.);
#8739=EDGE_CURVE('',#7109,#7111,#4004,.T.);
#8740=EDGE_CURVE('',#7142,#7142,#6596,.T.);
#8741=EDGE_CURVE('',#7137,#7139,#4005,.T.);
#8742=EDGE_CURVE('',#7140,#7136,#4006,.T.);
#8743=EDGE_CURVE('',#7064,#7143,#4007,.T.);
#8744=EDGE_CURVE('',#7143,#7144,#323,.T.);
#8745=EDGE_CURVE('',#7065,#7144,#4008,.T.);
#8746=EDGE_CURVE('',#7074,#7145,#4009,.T.);
#8747=EDGE_CURVE('',#7145,#7143,#324,.T.);
#8748=EDGE_CURVE('',#7073,#7146,#4010,.T.);
#8749=EDGE_CURVE('',#7146,#7145,#325,.T.);
#8750=EDGE_CURVE('',#7072,#7147,#4011,.T.);
#8751=EDGE_CURVE('',#7147,#7146,#326,.T.);
#8752=EDGE_CURVE('',#7071,#7148,#4012,.T.);
#8753=EDGE_CURVE('',#7148,#7147,#327,.T.);
#8754=EDGE_CURVE('',#7070,#7149,#4013,.T.);
#8755=EDGE_CURVE('',#7149,#7148,#328,.T.);
#8756=EDGE_CURVE('',#7069,#7150,#4014,.T.);
#8757=EDGE_CURVE('',#7150,#7149,#329,.T.);
#8758=EDGE_CURVE('',#7068,#7151,#4015,.T.);
#8759=EDGE_CURVE('',#7151,#7150,#330,.T.);
#8760=EDGE_CURVE('',#7067,#7152,#4016,.T.);
#8761=EDGE_CURVE('',#7152,#7151,#331,.T.);
#8762=EDGE_CURVE('',#7066,#7153,#4017,.T.);
#8763=EDGE_CURVE('',#7153,#7152,#332,.T.);
#8764=EDGE_CURVE('',#7144,#7153,#333,.T.);
#8765=EDGE_CURVE('',#7075,#7154,#4018,.T.);
#8766=EDGE_CURVE('',#7154,#7155,#4019,.T.);
#8767=EDGE_CURVE('',#7076,#7155,#4020,.T.);
#8768=EDGE_CURVE('',#7082,#7156,#4021,.T.);
#8769=EDGE_CURVE('',#7156,#7154,#4022,.T.);
#8770=EDGE_CURVE('',#7081,#7157,#4023,.T.);
#8771=EDGE_CURVE('',#7157,#7156,#4024,.T.);
#8772=EDGE_CURVE('',#7080,#7158,#4025,.T.);
#8773=EDGE_CURVE('',#7158,#7157,#4026,.T.);
#8774=EDGE_CURVE('',#7079,#7159,#4027,.T.);
#8775=EDGE_CURVE('',#7159,#7158,#4028,.T.);
#8776=EDGE_CURVE('',#7078,#7160,#4029,.T.);
#8777=EDGE_CURVE('',#7160,#7159,#4030,.T.);
#8778=EDGE_CURVE('',#7077,#7161,#4031,.T.);
#8779=EDGE_CURVE('',#7161,#7160,#4032,.T.);
#8780=EDGE_CURVE('',#7155,#7161,#4033,.T.);
#8781=EDGE_CURVE('',#7083,#7162,#4034,.T.);
#8782=EDGE_CURVE('',#7162,#7163,#334,.T.);
#8783=EDGE_CURVE('',#7084,#7163,#4035,.T.);
#8784=EDGE_CURVE('',#7098,#7164,#4036,.T.);
#8785=EDGE_CURVE('',#7164,#7162,#335,.T.);
#8786=EDGE_CURVE('',#7097,#7165,#4037,.T.);
#8787=EDGE_CURVE('',#7165,#7164,#336,.T.);
#8788=EDGE_CURVE('',#7096,#7166,#4038,.T.);
#8789=EDGE_CURVE('',#7166,#7165,#337,.T.);
#8790=EDGE_CURVE('',#7095,#7167,#4039,.T.);
#8791=EDGE_CURVE('',#7167,#7166,#338,.T.);
#8792=EDGE_CURVE('',#7094,#7168,#4040,.T.);
#8793=EDGE_CURVE('',#7168,#7167,#339,.T.);
#8794=EDGE_CURVE('',#7093,#7169,#4041,.T.);
#8795=EDGE_CURVE('',#7169,#7168,#340,.T.);
#8796=EDGE_CURVE('',#7092,#7170,#4042,.T.);
#8797=EDGE_CURVE('',#7170,#7169,#341,.T.);
#8798=EDGE_CURVE('',#7091,#7171,#4043,.T.);
#8799=EDGE_CURVE('',#7171,#7170,#342,.T.);
#8800=EDGE_CURVE('',#7090,#7172,#4044,.T.);
#8801=EDGE_CURVE('',#7172,#7171,#343,.T.);
#8802=EDGE_CURVE('',#7089,#7173,#4045,.T.);
#8803=EDGE_CURVE('',#7173,#7172,#344,.T.);
#8804=EDGE_CURVE('',#7088,#7174,#4046,.T.);
#8805=EDGE_CURVE('',#7174,#7173,#345,.T.);
#8806=EDGE_CURVE('',#7087,#7175,#4047,.T.);
#8807=EDGE_CURVE('',#7175,#7174,#346,.T.);
#8808=EDGE_CURVE('',#7086,#7176,#4048,.T.);
#8809=EDGE_CURVE('',#7176,#7175,#347,.T.);
#8810=EDGE_CURVE('',#7085,#7177,#4049,.T.);
#8811=EDGE_CURVE('',#7177,#7176,#348,.T.);
#8812=EDGE_CURVE('',#7163,#7177,#349,.T.);
#8813=EDGE_CURVE('',#7099,#7178,#4050,.T.);
#8814=EDGE_CURVE('',#7178,#7179,#4051,.T.);
#8815=EDGE_CURVE('',#7100,#7179,#4052,.T.);
#8816=EDGE_CURVE('',#7108,#7180,#4053,.T.);
#8817=EDGE_CURVE('',#7180,#7178,#4054,.T.);
#8818=EDGE_CURVE('',#7107,#7181,#4055,.T.);
#8819=EDGE_CURVE('',#7181,#7180,#4056,.T.);
#8820=EDGE_CURVE('',#7106,#7182,#4057,.T.);
#8821=EDGE_CURVE('',#7182,#7181,#4058,.T.);
#8822=EDGE_CURVE('',#7105,#7183,#4059,.T.);
#8823=EDGE_CURVE('',#7183,#7182,#4060,.T.);
#8824=EDGE_CURVE('',#7104,#7184,#4061,.T.);
#8825=EDGE_CURVE('',#7184,#7183,#4062,.T.);
#8826=EDGE_CURVE('',#7103,#7185,#4063,.T.);
#8827=EDGE_CURVE('',#7185,#7184,#4064,.T.);
#8828=EDGE_CURVE('',#7102,#7186,#4065,.T.);
#8829=EDGE_CURVE('',#7186,#7185,#4066,.T.);
#8830=EDGE_CURVE('',#7101,#7187,#4067,.T.);
#8831=EDGE_CURVE('',#7187,#7186,#4068,.T.);
#8832=EDGE_CURVE('',#7179,#7187,#4069,.T.);
#8833=EDGE_CURVE('',#7142,#7188,#4070,.T.);
#8834=EDGE_CURVE('',#7188,#7188,#6597,.T.);
#8835=EDGE_CURVE('',#7189,#7189,#6598,.T.);
#8836=EDGE_CURVE('',#7189,#7130,#4071,.T.);
#8837=EDGE_CURVE('',#6967,#7189,#4072,.T.);
#10802=ORIENTED_EDGE('',*,*,#8464,.T.);
#10803=ORIENTED_EDGE('',*,*,#8465,.T.);
#10804=ORIENTED_EDGE('',*,*,#8466,.T.);
#10805=ORIENTED_EDGE('',*,*,#8467,.T.);
#10806=ORIENTED_EDGE('',*,*,#8466,.F.);
#10807=ORIENTED_EDGE('',*,*,#8468,.F.);
#10808=ORIENTED_EDGE('',*,*,#8469,.T.);
#10809=ORIENTED_EDGE('',*,*,#8464,.F.);
#10810=ORIENTED_EDGE('',*,*,#8465,.F.);
#10811=ORIENTED_EDGE('',*,*,#8469,.F.);
#10812=ORIENTED_EDGE('',*,*,#8470,.T.);
#10813=ORIENTED_EDGE('',*,*,#8467,.F.);
#10814=ORIENTED_EDGE('',*,*,#8471,.T.);
#10815=ORIENTED_EDGE('',*,*,#8472,.T.);
#10816=ORIENTED_EDGE('',*,*,#8468,.T.);
#10817=ORIENTED_EDGE('',*,*,#8472,.F.);
#10818=ORIENTED_EDGE('',*,*,#8473,.F.);
#10819=ORIENTED_EDGE('',*,*,#8474,.F.);
#10820=ORIENTED_EDGE('',*,*,#8475,.F.);
#10821=ORIENTED_EDGE('',*,*,#8476,.F.);
#10822=ORIENTED_EDGE('',*,*,#8477,.F.);
#10823=ORIENTED_EDGE('',*,*,#8478,.F.);
#10824=ORIENTED_EDGE('',*,*,#8479,.F.);
#10825=ORIENTED_EDGE('',*,*,#8480,.F.);
#10826=ORIENTED_EDGE('',*,*,#8481,.F.);
#10827=ORIENTED_EDGE('',*,*,#8482,.F.);
#10828=ORIENTED_EDGE('',*,*,#8471,.F.);
#10829=ORIENTED_EDGE('',*,*,#8483,.T.);
#10830=ORIENTED_EDGE('',*,*,#8484,.F.);
#10831=ORIENTED_EDGE('',*,*,#8485,.T.);
#10832=ORIENTED_EDGE('',*,*,#8486,.T.);
#10833=ORIENTED_EDGE('',*,*,#8484,.T.);
#10834=ORIENTED_EDGE('',*,*,#8487,.T.);
#10835=ORIENTED_EDGE('',*,*,#8488,.T.);
#10836=ORIENTED_EDGE('',*,*,#8489,.T.);
#10837=ORIENTED_EDGE('',*,*,#8490,.T.);
#10838=ORIENTED_EDGE('',*,*,#8491,.T.);
#10839=ORIENTED_EDGE('',*,*,#8488,.F.);
#10840=ORIENTED_EDGE('',*,*,#8492,.T.);
#10841=ORIENTED_EDGE('',*,*,#8486,.F.);
#10842=ORIENTED_EDGE('',*,*,#8493,.F.);
#10843=ORIENTED_EDGE('',*,*,#8494,.F.);
#10844=ORIENTED_EDGE('',*,*,#8495,.F.);
#10845=ORIENTED_EDGE('',*,*,#8496,.F.);
#10846=ORIENTED_EDGE('',*,*,#8497,.F.);
#10847=ORIENTED_EDGE('',*,*,#8498,.F.);
#10848=ORIENTED_EDGE('',*,*,#8499,.F.);
#10849=ORIENTED_EDGE('',*,*,#8500,.F.);
#10850=ORIENTED_EDGE('',*,*,#8501,.F.);
#10851=ORIENTED_EDGE('',*,*,#8502,.F.);
#10852=ORIENTED_EDGE('',*,*,#8503,.F.);
#10853=ORIENTED_EDGE('',*,*,#8504,.T.);
#10854=ORIENTED_EDGE('',*,*,#8505,.F.);
#10855=ORIENTED_EDGE('',*,*,#8485,.F.);
#10856=ORIENTED_EDGE('',*,*,#8489,.F.);
#10857=ORIENTED_EDGE('',*,*,#8506,.T.);
#10858=ORIENTED_EDGE('',*,*,#8507,.F.);
#10859=ORIENTED_EDGE('',*,*,#8493,.T.);
#10860=ORIENTED_EDGE('',*,*,#8491,.F.);
#10861=ORIENTED_EDGE('',*,*,#8508,.T.);
#10862=ORIENTED_EDGE('',*,*,#8509,.F.);
#10863=ORIENTED_EDGE('',*,*,#8510,.F.);
#10864=ORIENTED_EDGE('',*,*,#8511,.F.);
#10865=ORIENTED_EDGE('',*,*,#8506,.F.);
#10866=ORIENTED_EDGE('',*,*,#8512,.T.);
#10867=ORIENTED_EDGE('',*,*,#8513,.F.);
#10868=ORIENTED_EDGE('',*,*,#8514,.T.);
#10869=ORIENTED_EDGE('',*,*,#8515,.T.);
#10870=ORIENTED_EDGE('',*,*,#8516,.T.);
#10871=ORIENTED_EDGE('',*,*,#8517,.F.);
#10872=ORIENTED_EDGE('',*,*,#8518,.T.);
#10873=ORIENTED_EDGE('',*,*,#8519,.T.);
#10874=ORIENTED_EDGE('',*,*,#8517,.T.);
#10875=ORIENTED_EDGE('',*,*,#8520,.T.);
#10876=ORIENTED_EDGE('',*,*,#8521,.T.);
#10877=ORIENTED_EDGE('',*,*,#8522,.T.);
#10878=ORIENTED_EDGE('',*,*,#8523,.T.);
#10879=ORIENTED_EDGE('',*,*,#8524,.T.);
#10880=ORIENTED_EDGE('',*,*,#8525,.T.);
#10881=ORIENTED_EDGE('',*,*,#8526,.T.);
#10882=ORIENTED_EDGE('',*,*,#8525,.F.);
#10883=ORIENTED_EDGE('',*,*,#8527,.T.);
#10884=ORIENTED_EDGE('',*,*,#8521,.F.);
#10885=ORIENTED_EDGE('',*,*,#8528,.T.);
#10886=ORIENTED_EDGE('',*,*,#8529,.T.);
#10887=ORIENTED_EDGE('',*,*,#8530,.T.);
#10888=ORIENTED_EDGE('',*,*,#8531,.T.);
#10889=ORIENTED_EDGE('',*,*,#8532,.T.);
#10890=ORIENTED_EDGE('',*,*,#8529,.F.);
#10891=ORIENTED_EDGE('',*,*,#8533,.T.);
#10892=ORIENTED_EDGE('',*,*,#8523,.F.);
#10893=ORIENTED_EDGE('',*,*,#8534,.T.);
#10894=ORIENTED_EDGE('',*,*,#8535,.T.);
#10895=ORIENTED_EDGE('',*,*,#8536,.T.);
#10896=ORIENTED_EDGE('',*,*,#8537,.T.);
#10897=ORIENTED_EDGE('',*,*,#8538,.T.);
#10898=ORIENTED_EDGE('',*,*,#8535,.F.);
#10899=ORIENTED_EDGE('',*,*,#8539,.T.);
#10900=ORIENTED_EDGE('',*,*,#8531,.F.);
#10901=ORIENTED_EDGE('',*,*,#8540,.T.);
#10902=ORIENTED_EDGE('',*,*,#8513,.T.);
#10903=ORIENTED_EDGE('',*,*,#8541,.T.);
#10904=ORIENTED_EDGE('',*,*,#8542,.T.);
#10905=ORIENTED_EDGE('',*,*,#8543,.T.);
#10906=ORIENTED_EDGE('',*,*,#8542,.F.);
#10907=ORIENTED_EDGE('',*,*,#8544,.T.);
#10908=ORIENTED_EDGE('',*,*,#8537,.F.);
#10909=ORIENTED_EDGE('',*,*,#8545,.T.);
#10910=ORIENTED_EDGE('',*,*,#8526,.F.);
#10911=ORIENTED_EDGE('',*,*,#8528,.F.);
#10912=ORIENTED_EDGE('',*,*,#8520,.F.);
#10913=ORIENTED_EDGE('',*,*,#8516,.F.);
#10914=ORIENTED_EDGE('',*,*,#8546,.T.);
#10915=ORIENTED_EDGE('',*,*,#8547,.T.);
#10916=ORIENTED_EDGE('',*,*,#8548,.T.);
#10917=ORIENTED_EDGE('',*,*,#8519,.F.);
#10918=ORIENTED_EDGE('',*,*,#8549,.F.);
#10919=ORIENTED_EDGE('',*,*,#8550,.F.);
#10920=ORIENTED_EDGE('',*,*,#8551,.F.);
#10921=ORIENTED_EDGE('',*,*,#8546,.F.);
#10922=ORIENTED_EDGE('',*,*,#8518,.F.);
#10923=ORIENTED_EDGE('',*,*,#8522,.F.);
#10924=ORIENTED_EDGE('',*,*,#8552,.T.);
#10925=ORIENTED_EDGE('',*,*,#8553,.T.);
#10926=ORIENTED_EDGE('',*,*,#8549,.T.);
#10927=ORIENTED_EDGE('',*,*,#8527,.F.);
#10928=ORIENTED_EDGE('',*,*,#8524,.F.);
#10929=ORIENTED_EDGE('',*,*,#8533,.F.);
#10930=ORIENTED_EDGE('',*,*,#8532,.F.);
#10931=ORIENTED_EDGE('',*,*,#8539,.F.);
#10932=ORIENTED_EDGE('',*,*,#8538,.F.);
#10933=ORIENTED_EDGE('',*,*,#8544,.F.);
#10934=ORIENTED_EDGE('',*,*,#8554,.F.);
#10935=ORIENTED_EDGE('',*,*,#8555,.F.);
#10936=ORIENTED_EDGE('',*,*,#8552,.F.);
#10937=ORIENTED_EDGE('',*,*,#8556,.T.);
#10938=ORIENTED_EDGE('',*,*,#8557,.T.);
#10939=ORIENTED_EDGE('',*,*,#8558,.T.);
#10940=ORIENTED_EDGE('',*,*,#8559,.T.);
#10941=ORIENTED_EDGE('',*,*,#8558,.F.);
#10942=ORIENTED_EDGE('',*,*,#8560,.T.);
#10943=ORIENTED_EDGE('',*,*,#8561,.T.);
#10944=ORIENTED_EDGE('',*,*,#8556,.F.);
#10945=ORIENTED_EDGE('',*,*,#8562,.T.);
#10946=ORIENTED_EDGE('',*,*,#8563,.T.);
#10947=ORIENTED_EDGE('',*,*,#8561,.F.);
#10948=ORIENTED_EDGE('',*,*,#8564,.T.);
#10949=ORIENTED_EDGE('',*,*,#8565,.T.);
#10950=ORIENTED_EDGE('',*,*,#8566,.T.);
#10951=ORIENTED_EDGE('',*,*,#8560,.F.);
#10952=ORIENTED_EDGE('',*,*,#8567,.T.);
#10953=ORIENTED_EDGE('',*,*,#8568,.T.);
#10954=ORIENTED_EDGE('',*,*,#8569,.T.);
#10955=ORIENTED_EDGE('',*,*,#8557,.F.);
#10956=ORIENTED_EDGE('',*,*,#8570,.F.);
#10957=ORIENTED_EDGE('',*,*,#8571,.T.);
#10958=ORIENTED_EDGE('',*,*,#8567,.F.);
#10959=ORIENTED_EDGE('',*,*,#8572,.F.);
#10960=ORIENTED_EDGE('',*,*,#8573,.F.);
#10961=ORIENTED_EDGE('',*,*,#8574,.F.);
#10962=ORIENTED_EDGE('',*,*,#8575,.T.);
#10963=ORIENTED_EDGE('',*,*,#8576,.T.);
#10964=ORIENTED_EDGE('',*,*,#8573,.T.);
#10965=ORIENTED_EDGE('',*,*,#8509,.T.);
#10966=ORIENTED_EDGE('',*,*,#8577,.T.);
#10967=ORIENTED_EDGE('',*,*,#8578,.T.);
#10968=ORIENTED_EDGE('',*,*,#8574,.T.);
#10969=ORIENTED_EDGE('',*,*,#8579,.T.);
#10970=ORIENTED_EDGE('',*,*,#8580,.F.);
#10971=ORIENTED_EDGE('',*,*,#8581,.F.);
#10972=ORIENTED_EDGE('',*,*,#8582,.F.);
#10973=ORIENTED_EDGE('',*,*,#8583,.T.);
#10974=ORIENTED_EDGE('',*,*,#8584,.T.);
#10975=ORIENTED_EDGE('',*,*,#8507,.T.);
#10976=ORIENTED_EDGE('',*,*,#8583,.F.);
#10977=ORIENTED_EDGE('',*,*,#8511,.T.);
#10978=ORIENTED_EDGE('',*,*,#8581,.T.);
#10979=ORIENTED_EDGE('',*,*,#8585,.T.);
#10980=ORIENTED_EDGE('',*,*,#8572,.T.);
#10981=ORIENTED_EDGE('',*,*,#8586,.T.);
#10982=ORIENTED_EDGE('',*,*,#8582,.T.);
#10983=ORIENTED_EDGE('',*,*,#8510,.T.);
#10984=ORIENTED_EDGE('',*,*,#8587,.F.);
#10985=ORIENTED_EDGE('',*,*,#8588,.F.);
#10986=ORIENTED_EDGE('',*,*,#8589,.F.);
#10987=ORIENTED_EDGE('',*,*,#8590,.T.);
#10988=ORIENTED_EDGE('',*,*,#8591,.T.);
#10989=ORIENTED_EDGE('',*,*,#8592,.T.);
#10990=ORIENTED_EDGE('',*,*,#8590,.F.);
#10991=ORIENTED_EDGE('',*,*,#8593,.T.);
#10992=ORIENTED_EDGE('',*,*,#8588,.T.);
#10993=ORIENTED_EDGE('',*,*,#8594,.T.);
#10994=ORIENTED_EDGE('',*,*,#8580,.T.);
#10995=ORIENTED_EDGE('',*,*,#8595,.T.);
#10996=ORIENTED_EDGE('',*,*,#8589,.T.);
#10997=ORIENTED_EDGE('',*,*,#8596,.T.);
#10998=ORIENTED_EDGE('',*,*,#8547,.F.);
#10999=ORIENTED_EDGE('',*,*,#8597,.F.);
#11000=ORIENTED_EDGE('',*,*,#8598,.F.);
#11001=ORIENTED_EDGE('',*,*,#8599,.T.);
#11002=ORIENTED_EDGE('',*,*,#8600,.T.);
#11003=ORIENTED_EDGE('',*,*,#8601,.T.);
#11004=ORIENTED_EDGE('',*,*,#8599,.F.);
#11005=ORIENTED_EDGE('',*,*,#8602,.T.);
#11006=ORIENTED_EDGE('',*,*,#8597,.T.);
#11007=ORIENTED_EDGE('',*,*,#8551,.T.);
#11008=ORIENTED_EDGE('',*,*,#8587,.T.);
#11009=ORIENTED_EDGE('',*,*,#8603,.T.);
#11010=ORIENTED_EDGE('',*,*,#8598,.T.);
#11011=ORIENTED_EDGE('',*,*,#8604,.T.);
#11012=ORIENTED_EDGE('',*,*,#8605,.F.);
#11013=ORIENTED_EDGE('',*,*,#8606,.F.);
#11014=ORIENTED_EDGE('',*,*,#8607,.F.);
#11015=ORIENTED_EDGE('',*,*,#8608,.T.);
#11016=ORIENTED_EDGE('',*,*,#8498,.T.);
#11017=ORIENTED_EDGE('',*,*,#8606,.T.);
#11018=ORIENTED_EDGE('',*,*,#8609,.T.);
#11019=ORIENTED_EDGE('',*,*,#8608,.F.);
#11020=ORIENTED_EDGE('',*,*,#8610,.T.);
#11021=ORIENTED_EDGE('',*,*,#8611,.T.);
#11022=ORIENTED_EDGE('',*,*,#8612,.T.);
#11023=ORIENTED_EDGE('',*,*,#8555,.T.);
#11024=ORIENTED_EDGE('',*,*,#8607,.T.);
#11025=ORIENTED_EDGE('',*,*,#8497,.T.);
#11026=ORIENTED_EDGE('',*,*,#8512,.F.);
#11027=ORIENTED_EDGE('',*,*,#8613,.T.);
#11028=ORIENTED_EDGE('',*,*,#8605,.T.);
#11029=ORIENTED_EDGE('',*,*,#8554,.T.);
#11030=ORIENTED_EDGE('',*,*,#8541,.F.);
#11031=ORIENTED_EDGE('',*,*,#8614,.T.);
#11032=ORIENTED_EDGE('',*,*,#8615,.T.);
#11033=ORIENTED_EDGE('',*,*,#8616,.T.);
#11034=ORIENTED_EDGE('',*,*,#8536,.F.);
#11035=ORIENTED_EDGE('',*,*,#8617,.T.);
#11036=ORIENTED_EDGE('',*,*,#8614,.F.);
#11037=ORIENTED_EDGE('',*,*,#8618,.T.);
#11038=ORIENTED_EDGE('',*,*,#8514,.F.);
#11039=ORIENTED_EDGE('',*,*,#8543,.F.);
#11040=ORIENTED_EDGE('',*,*,#8545,.F.);
#11041=ORIENTED_EDGE('',*,*,#8612,.F.);
#11042=ORIENTED_EDGE('',*,*,#8619,.T.);
#11043=ORIENTED_EDGE('',*,*,#8553,.F.);
#11044=ORIENTED_EDGE('',*,*,#8585,.F.);
#11045=ORIENTED_EDGE('',*,*,#8596,.F.);
#11046=ORIENTED_EDGE('',*,*,#8593,.F.);
#11047=ORIENTED_EDGE('',*,*,#8620,.F.);
#11048=ORIENTED_EDGE('',*,*,#8621,.T.);
#11049=ORIENTED_EDGE('',*,*,#8622,.T.);
#11050=ORIENTED_EDGE('',*,*,#8623,.T.);
#11051=ORIENTED_EDGE('',*,*,#8624,.T.);
#11052=ORIENTED_EDGE('',*,*,#8625,.T.);
#11053=ORIENTED_EDGE('',*,*,#8626,.T.);
#11054=ORIENTED_EDGE('',*,*,#8627,.T.);
#11055=ORIENTED_EDGE('',*,*,#8628,.T.);
#11056=ORIENTED_EDGE('',*,*,#8629,.T.);
#11057=ORIENTED_EDGE('',*,*,#8630,.T.);
#11058=ORIENTED_EDGE('',*,*,#8631,.T.);
#11059=ORIENTED_EDGE('',*,*,#8632,.T.);
#11060=ORIENTED_EDGE('',*,*,#8633,.T.);
#11061=ORIENTED_EDGE('',*,*,#8634,.T.);
#11062=ORIENTED_EDGE('',*,*,#8635,.T.);
#11063=ORIENTED_EDGE('',*,*,#8636,.T.);
#11064=ORIENTED_EDGE('',*,*,#8637,.T.);
#11065=ORIENTED_EDGE('',*,*,#8638,.T.);
#11066=ORIENTED_EDGE('',*,*,#8639,.T.);
#11067=ORIENTED_EDGE('',*,*,#8640,.T.);
#11068=ORIENTED_EDGE('',*,*,#8641,.T.);
#11069=ORIENTED_EDGE('',*,*,#8642,.T.);
#11070=ORIENTED_EDGE('',*,*,#8643,.T.);
#11071=ORIENTED_EDGE('',*,*,#8644,.T.);
#11072=ORIENTED_EDGE('',*,*,#8645,.T.);
#11073=ORIENTED_EDGE('',*,*,#8646,.T.);
#11074=ORIENTED_EDGE('',*,*,#8647,.T.);
#11075=ORIENTED_EDGE('',*,*,#8648,.T.);
#11076=ORIENTED_EDGE('',*,*,#8649,.T.);
#11077=ORIENTED_EDGE('',*,*,#8650,.T.);
#11078=ORIENTED_EDGE('',*,*,#8651,.T.);
#11079=ORIENTED_EDGE('',*,*,#8652,.T.);
#11080=ORIENTED_EDGE('',*,*,#8653,.T.);
#11081=ORIENTED_EDGE('',*,*,#8654,.T.);
#11082=ORIENTED_EDGE('',*,*,#8655,.T.);
#11083=ORIENTED_EDGE('',*,*,#8656,.T.);
#11084=ORIENTED_EDGE('',*,*,#8657,.T.);
#11085=ORIENTED_EDGE('',*,*,#8658,.T.);
#11086=ORIENTED_EDGE('',*,*,#8659,.T.);
#11087=ORIENTED_EDGE('',*,*,#8660,.T.);
#11088=ORIENTED_EDGE('',*,*,#8661,.T.);
#11089=ORIENTED_EDGE('',*,*,#8662,.T.);
#11090=ORIENTED_EDGE('',*,*,#8663,.T.);
#11091=ORIENTED_EDGE('',*,*,#8664,.T.);
#11092=ORIENTED_EDGE('',*,*,#8665,.T.);
#11093=ORIENTED_EDGE('',*,*,#8594,.F.);
#11094=ORIENTED_EDGE('',*,*,#8604,.F.);
#11095=ORIENTED_EDGE('',*,*,#8602,.F.);
#11096=ORIENTED_EDGE('',*,*,#8666,.F.);
#11097=ORIENTED_EDGE('',*,*,#8591,.F.);
#11098=ORIENTED_EDGE('',*,*,#8666,.T.);
#11099=ORIENTED_EDGE('',*,*,#8601,.F.);
#11100=ORIENTED_EDGE('',*,*,#8495,.T.);
#11101=ORIENTED_EDGE('',*,*,#8600,.F.);
#11102=ORIENTED_EDGE('',*,*,#8550,.T.);
#11103=ORIENTED_EDGE('',*,*,#8619,.F.);
#11104=ORIENTED_EDGE('',*,*,#8496,.T.);
#11105=ORIENTED_EDGE('',*,*,#8611,.F.);
#11106=ORIENTED_EDGE('',*,*,#8667,.T.);
#11107=ORIENTED_EDGE('',*,*,#8668,.F.);
#11108=ORIENTED_EDGE('',*,*,#8499,.T.);
#11109=ORIENTED_EDGE('',*,*,#8515,.F.);
#11110=ORIENTED_EDGE('',*,*,#8618,.F.);
#11111=ORIENTED_EDGE('',*,*,#8669,.F.);
#11112=ORIENTED_EDGE('',*,*,#8609,.F.);
#11113=ORIENTED_EDGE('',*,*,#8613,.F.);
#11114=ORIENTED_EDGE('',*,*,#8610,.F.);
#11115=ORIENTED_EDGE('',*,*,#8669,.T.);
#11116=ORIENTED_EDGE('',*,*,#8616,.F.);
#11117=ORIENTED_EDGE('',*,*,#8670,.T.);
#11118=ORIENTED_EDGE('',*,*,#8615,.F.);
#11119=ORIENTED_EDGE('',*,*,#8671,.T.);
#11120=ORIENTED_EDGE('',*,*,#8672,.F.);
#11121=ORIENTED_EDGE('',*,*,#8673,.T.);
#11122=ORIENTED_EDGE('',*,*,#8584,.F.);
#11123=ORIENTED_EDGE('',*,*,#8620,.T.);
#11124=ORIENTED_EDGE('',*,*,#8592,.F.);
#11125=ORIENTED_EDGE('',*,*,#8494,.T.);
#11126=ORIENTED_EDGE('',*,*,#8483,.F.);
#11127=ORIENTED_EDGE('',*,*,#8505,.T.);
#11128=ORIENTED_EDGE('',*,*,#8674,.T.);
#11129=ORIENTED_EDGE('',*,*,#8675,.T.);
#11130=ORIENTED_EDGE('',*,*,#8487,.F.);
#11131=ORIENTED_EDGE('',*,*,#8492,.F.);
#11132=ORIENTED_EDGE('',*,*,#8675,.F.);
#11133=ORIENTED_EDGE('',*,*,#8676,.T.);
#11134=ORIENTED_EDGE('',*,*,#8564,.F.);
#11135=ORIENTED_EDGE('',*,*,#8569,.F.);
#11136=ORIENTED_EDGE('',*,*,#8677,.T.);
#11137=ORIENTED_EDGE('',*,*,#8562,.F.);
#11138=ORIENTED_EDGE('',*,*,#8678,.T.);
#11139=ORIENTED_EDGE('',*,*,#8679,.T.);
#11140=ORIENTED_EDGE('',*,*,#8482,.T.);
#11141=ORIENTED_EDGE('',*,*,#8563,.F.);
#11142=ORIENTED_EDGE('',*,*,#8481,.T.);
#11143=ORIENTED_EDGE('',*,*,#8680,.T.);
#11144=ORIENTED_EDGE('',*,*,#8570,.T.);
#11145=ORIENTED_EDGE('',*,*,#8559,.F.);
#11146=ORIENTED_EDGE('',*,*,#8566,.F.);
#11147=ORIENTED_EDGE('',*,*,#8681,.T.);
#11148=ORIENTED_EDGE('',*,*,#8678,.F.);
#11149=ORIENTED_EDGE('',*,*,#8682,.F.);
#11150=ORIENTED_EDGE('',*,*,#8683,.F.);
#11151=ORIENTED_EDGE('',*,*,#8684,.F.);
#11152=ORIENTED_EDGE('',*,*,#8685,.T.);
#11153=ORIENTED_EDGE('',*,*,#8479,.T.);
#11154=ORIENTED_EDGE('',*,*,#8683,.T.);
#11155=ORIENTED_EDGE('',*,*,#8686,.T.);
#11156=ORIENTED_EDGE('',*,*,#8687,.T.);
#11157=ORIENTED_EDGE('',*,*,#8688,.T.);
#11158=ORIENTED_EDGE('',*,*,#8684,.T.);
#11159=ORIENTED_EDGE('',*,*,#8478,.T.);
#11160=ORIENTED_EDGE('',*,*,#8689,.T.);
#11161=ORIENTED_EDGE('',*,*,#8690,.T.);
#11162=ORIENTED_EDGE('',*,*,#8691,.T.);
#11163=ORIENTED_EDGE('',*,*,#8689,.F.);
#11164=ORIENTED_EDGE('',*,*,#8692,.T.);
#11165=ORIENTED_EDGE('',*,*,#8682,.T.);
#11166=ORIENTED_EDGE('',*,*,#8693,.T.);
#11167=ORIENTED_EDGE('',*,*,#8686,.F.);
#11168=ORIENTED_EDGE('',*,*,#8692,.F.);
#11169=ORIENTED_EDGE('',*,*,#8694,.F.);
#11170=ORIENTED_EDGE('',*,*,#8695,.T.);
#11171=ORIENTED_EDGE('',*,*,#8691,.F.);
#11172=ORIENTED_EDGE('',*,*,#8696,.T.);
#11173=ORIENTED_EDGE('',*,*,#8697,.T.);
#11174=ORIENTED_EDGE('',*,*,#8694,.T.);
#11175=ORIENTED_EDGE('',*,*,#8690,.F.);
#11176=ORIENTED_EDGE('',*,*,#8698,.T.);
#11177=ORIENTED_EDGE('',*,*,#8699,.T.);
#11178=ORIENTED_EDGE('',*,*,#8700,.T.);
#11179=ORIENTED_EDGE('',*,*,#8696,.F.);
#11180=ORIENTED_EDGE('',*,*,#8700,.F.);
#11181=ORIENTED_EDGE('',*,*,#8701,.T.);
#11182=ORIENTED_EDGE('',*,*,#8702,.T.);
#11183=ORIENTED_EDGE('',*,*,#8703,.T.);
#11184=ORIENTED_EDGE('',*,*,#8704,.T.);
#11185=ORIENTED_EDGE('',*,*,#8705,.T.);
#11186=ORIENTED_EDGE('',*,*,#8703,.F.);
#11187=ORIENTED_EDGE('',*,*,#8705,.F.);
#11188=ORIENTED_EDGE('',*,*,#8706,.T.);
#11189=ORIENTED_EDGE('',*,*,#8707,.F.);
#11190=ORIENTED_EDGE('',*,*,#8708,.F.);
#11191=ORIENTED_EDGE('',*,*,#8706,.F.);
#11192=ORIENTED_EDGE('',*,*,#8704,.F.);
#11193=ORIENTED_EDGE('',*,*,#8702,.F.);
#11194=ORIENTED_EDGE('',*,*,#8709,.T.);
#11195=ORIENTED_EDGE('',*,*,#8707,.T.);
#11196=ORIENTED_EDGE('',*,*,#8708,.T.);
#11197=ORIENTED_EDGE('',*,*,#8710,.T.);
#11198=ORIENTED_EDGE('',*,*,#8711,.T.);
#11199=ORIENTED_EDGE('',*,*,#8712,.T.);
#11200=ORIENTED_EDGE('',*,*,#8710,.F.);
#11201=ORIENTED_EDGE('',*,*,#8712,.F.);
#11202=ORIENTED_EDGE('',*,*,#8713,.T.);
#11203=ORIENTED_EDGE('',*,*,#8714,.F.);
#11204=ORIENTED_EDGE('',*,*,#8681,.F.);
#11205=ORIENTED_EDGE('',*,*,#8565,.F.);
#11206=ORIENTED_EDGE('',*,*,#8677,.F.);
#11207=ORIENTED_EDGE('',*,*,#8568,.F.);
#11208=ORIENTED_EDGE('',*,*,#8571,.F.);
#11209=ORIENTED_EDGE('',*,*,#8715,.F.);
#11210=ORIENTED_EDGE('',*,*,#8695,.F.);
#11211=ORIENTED_EDGE('',*,*,#8697,.F.);
#11212=ORIENTED_EDGE('',*,*,#8701,.F.);
#11213=ORIENTED_EDGE('',*,*,#8699,.F.);
#11214=ORIENTED_EDGE('',*,*,#8716,.F.);
#11215=ORIENTED_EDGE('',*,*,#8717,.F.);
#11216=ORIENTED_EDGE('',*,*,#8718,.F.);
#11217=ORIENTED_EDGE('',*,*,#8577,.F.);
#11218=ORIENTED_EDGE('',*,*,#8719,.F.);
#11219=ORIENTED_EDGE('',*,*,#8575,.F.);
#11220=ORIENTED_EDGE('',*,*,#8508,.F.);
#11221=ORIENTED_EDGE('',*,*,#8490,.F.);
#11222=ORIENTED_EDGE('',*,*,#8676,.F.);
#11223=ORIENTED_EDGE('',*,*,#8674,.F.);
#11224=ORIENTED_EDGE('',*,*,#8504,.F.);
#11225=ORIENTED_EDGE('',*,*,#8720,.F.);
#11226=ORIENTED_EDGE('',*,*,#8713,.F.);
#11227=ORIENTED_EDGE('',*,*,#8711,.F.);
#11228=ORIENTED_EDGE('',*,*,#8480,.T.);
#11229=ORIENTED_EDGE('',*,*,#8685,.F.);
#11230=ORIENTED_EDGE('',*,*,#8715,.T.);
#11231=ORIENTED_EDGE('',*,*,#8680,.F.);
#11232=ORIENTED_EDGE('',*,*,#8721,.T.);
#11233=ORIENTED_EDGE('',*,*,#8722,.T.);
#11234=ORIENTED_EDGE('',*,*,#8723,.T.);
#11235=ORIENTED_EDGE('',*,*,#8724,.T.);
#11236=ORIENTED_EDGE('',*,*,#8672,.T.);
#11237=ORIENTED_EDGE('',*,*,#8725,.T.);
#11238=ORIENTED_EDGE('',*,*,#8723,.F.);
#11239=ORIENTED_EDGE('',*,*,#8726,.T.);
#11240=ORIENTED_EDGE('',*,*,#8727,.T.);
#11241=ORIENTED_EDGE('',*,*,#8728,.T.);
#11242=ORIENTED_EDGE('',*,*,#8729,.T.);
#11243=ORIENTED_EDGE('',*,*,#8501,.T.);
#11244=ORIENTED_EDGE('',*,*,#8730,.T.);
#11245=ORIENTED_EDGE('',*,*,#8502,.T.);
#11246=ORIENTED_EDGE('',*,*,#8729,.F.);
#11247=ORIENTED_EDGE('',*,*,#8731,.T.);
#11248=ORIENTED_EDGE('',*,*,#8503,.T.);
#11249=ORIENTED_EDGE('',*,*,#8730,.F.);
#11250=ORIENTED_EDGE('',*,*,#8474,.T.);
#11251=ORIENTED_EDGE('',*,*,#8732,.T.);
#11252=ORIENTED_EDGE('',*,*,#8668,.T.);
#11253=ORIENTED_EDGE('',*,*,#8733,.T.);
#11254=ORIENTED_EDGE('',*,*,#8727,.F.);
#11255=ORIENTED_EDGE('',*,*,#8500,.T.);
#11256=ORIENTED_EDGE('',*,*,#8473,.T.);
#11257=ORIENTED_EDGE('',*,*,#8679,.F.);
#11258=ORIENTED_EDGE('',*,*,#8714,.T.);
#11259=ORIENTED_EDGE('',*,*,#8720,.T.);
#11260=ORIENTED_EDGE('',*,*,#8732,.F.);
#11261=ORIENTED_EDGE('',*,*,#8734,.T.);
#11262=ORIENTED_EDGE('',*,*,#8735,.T.);
#11263=ORIENTED_EDGE('',*,*,#8721,.F.);
#11264=ORIENTED_EDGE('',*,*,#8736,.T.);
#11265=ORIENTED_EDGE('',*,*,#8476,.T.);
#11266=ORIENTED_EDGE('',*,*,#8734,.F.);
#11267=ORIENTED_EDGE('',*,*,#8737,.T.);
#11268=ORIENTED_EDGE('',*,*,#8738,.T.);
#11269=ORIENTED_EDGE('',*,*,#8717,.T.);
#11270=ORIENTED_EDGE('',*,*,#8687,.F.);
#11271=ORIENTED_EDGE('',*,*,#8477,.T.);
#11272=ORIENTED_EDGE('',*,*,#8738,.F.);
#11273=ORIENTED_EDGE('',*,*,#8667,.F.);
#11274=ORIENTED_EDGE('',*,*,#8670,.F.);
#11275=ORIENTED_EDGE('',*,*,#8673,.F.);
#11276=ORIENTED_EDGE('',*,*,#8739,.F.);
#11277=ORIENTED_EDGE('',*,*,#8740,.T.);
#11278=ORIENTED_EDGE('',*,*,#8733,.F.);
#11279=ORIENTED_EDGE('',*,*,#8739,.T.);
#11280=ORIENTED_EDGE('',*,*,#8726,.F.);
#11281=ORIENTED_EDGE('',*,*,#8741,.T.);
#11282=ORIENTED_EDGE('',*,*,#8728,.F.);
#11283=ORIENTED_EDGE('',*,*,#8741,.F.);
#11284=ORIENTED_EDGE('',*,*,#8722,.F.);
#11285=ORIENTED_EDGE('',*,*,#8742,.F.);
#11286=ORIENTED_EDGE('',*,*,#8731,.F.);
#11287=ORIENTED_EDGE('',*,*,#8742,.T.);
#11288=ORIENTED_EDGE('',*,*,#8735,.F.);
#11289=ORIENTED_EDGE('',*,*,#8475,.T.);
#11290=ORIENTED_EDGE('',*,*,#8621,.F.);
#11291=ORIENTED_EDGE('',*,*,#8743,.T.);
#11292=ORIENTED_EDGE('',*,*,#8744,.T.);
#11293=ORIENTED_EDGE('',*,*,#8745,.F.);
#11294=ORIENTED_EDGE('',*,*,#8631,.F.);
#11295=ORIENTED_EDGE('',*,*,#8746,.T.);
#11296=ORIENTED_EDGE('',*,*,#8747,.T.);
#11297=ORIENTED_EDGE('',*,*,#8743,.F.);
#11298=ORIENTED_EDGE('',*,*,#8630,.F.);
#11299=ORIENTED_EDGE('',*,*,#8748,.T.);
#11300=ORIENTED_EDGE('',*,*,#8749,.T.);
#11301=ORIENTED_EDGE('',*,*,#8746,.F.);
#11302=ORIENTED_EDGE('',*,*,#8629,.F.);
#11303=ORIENTED_EDGE('',*,*,#8750,.T.);
#11304=ORIENTED_EDGE('',*,*,#8751,.T.);
#11305=ORIENTED_EDGE('',*,*,#8748,.F.);
#11306=ORIENTED_EDGE('',*,*,#8628,.F.);
#11307=ORIENTED_EDGE('',*,*,#8752,.T.);
#11308=ORIENTED_EDGE('',*,*,#8753,.T.);
#11309=ORIENTED_EDGE('',*,*,#8750,.F.);
#11310=ORIENTED_EDGE('',*,*,#8627,.F.);
#11311=ORIENTED_EDGE('',*,*,#8754,.T.);
#11312=ORIENTED_EDGE('',*,*,#8755,.T.);
#11313=ORIENTED_EDGE('',*,*,#8752,.F.);
#11314=ORIENTED_EDGE('',*,*,#8626,.F.);
#11315=ORIENTED_EDGE('',*,*,#8756,.T.);
#11316=ORIENTED_EDGE('',*,*,#8757,.T.);
#11317=ORIENTED_EDGE('',*,*,#8754,.F.);
#11318=ORIENTED_EDGE('',*,*,#8625,.F.);
#11319=ORIENTED_EDGE('',*,*,#8758,.T.);
#11320=ORIENTED_EDGE('',*,*,#8759,.T.);
#11321=ORIENTED_EDGE('',*,*,#8756,.F.);
#11322=ORIENTED_EDGE('',*,*,#8624,.F.);
#11323=ORIENTED_EDGE('',*,*,#8760,.T.);
#11324=ORIENTED_EDGE('',*,*,#8761,.T.);
#11325=ORIENTED_EDGE('',*,*,#8758,.F.);
#11326=ORIENTED_EDGE('',*,*,#8623,.F.);
#11327=ORIENTED_EDGE('',*,*,#8762,.T.);
#11328=ORIENTED_EDGE('',*,*,#8763,.T.);
#11329=ORIENTED_EDGE('',*,*,#8760,.F.);
#11330=ORIENTED_EDGE('',*,*,#8622,.F.);
#11331=ORIENTED_EDGE('',*,*,#8745,.T.);
#11332=ORIENTED_EDGE('',*,*,#8764,.T.);
#11333=ORIENTED_EDGE('',*,*,#8762,.F.);
#11334=ORIENTED_EDGE('',*,*,#8764,.F.);
#11335=ORIENTED_EDGE('',*,*,#8744,.F.);
#11336=ORIENTED_EDGE('',*,*,#8747,.F.);
#11337=ORIENTED_EDGE('',*,*,#8749,.F.);
#11338=ORIENTED_EDGE('',*,*,#8751,.F.);
#11339=ORIENTED_EDGE('',*,*,#8753,.F.);
#11340=ORIENTED_EDGE('',*,*,#8755,.F.);
#11341=ORIENTED_EDGE('',*,*,#8757,.F.);
#11342=ORIENTED_EDGE('',*,*,#8759,.F.);
#11343=ORIENTED_EDGE('',*,*,#8761,.F.);
#11344=ORIENTED_EDGE('',*,*,#8763,.F.);
#11345=ORIENTED_EDGE('',*,*,#8632,.F.);
#11346=ORIENTED_EDGE('',*,*,#8765,.T.);
#11347=ORIENTED_EDGE('',*,*,#8766,.T.);
#11348=ORIENTED_EDGE('',*,*,#8767,.F.);
#11349=ORIENTED_EDGE('',*,*,#8639,.F.);
#11350=ORIENTED_EDGE('',*,*,#8768,.T.);
#11351=ORIENTED_EDGE('',*,*,#8769,.T.);
#11352=ORIENTED_EDGE('',*,*,#8765,.F.);
#11353=ORIENTED_EDGE('',*,*,#8638,.F.);
#11354=ORIENTED_EDGE('',*,*,#8770,.T.);
#11355=ORIENTED_EDGE('',*,*,#8771,.T.);
#11356=ORIENTED_EDGE('',*,*,#8768,.F.);
#11357=ORIENTED_EDGE('',*,*,#8637,.F.);
#11358=ORIENTED_EDGE('',*,*,#8772,.T.);
#11359=ORIENTED_EDGE('',*,*,#8773,.T.);
#11360=ORIENTED_EDGE('',*,*,#8770,.F.);
#11361=ORIENTED_EDGE('',*,*,#8636,.F.);
#11362=ORIENTED_EDGE('',*,*,#8774,.T.);
#11363=ORIENTED_EDGE('',*,*,#8775,.T.);
#11364=ORIENTED_EDGE('',*,*,#8772,.F.);
#11365=ORIENTED_EDGE('',*,*,#8635,.F.);
#11366=ORIENTED_EDGE('',*,*,#8776,.T.);
#11367=ORIENTED_EDGE('',*,*,#8777,.T.);
#11368=ORIENTED_EDGE('',*,*,#8774,.F.);
#11369=ORIENTED_EDGE('',*,*,#8634,.F.);
#11370=ORIENTED_EDGE('',*,*,#8778,.T.);
#11371=ORIENTED_EDGE('',*,*,#8779,.T.);
#11372=ORIENTED_EDGE('',*,*,#8776,.F.);
#11373=ORIENTED_EDGE('',*,*,#8633,.F.);
#11374=ORIENTED_EDGE('',*,*,#8767,.T.);
#11375=ORIENTED_EDGE('',*,*,#8780,.T.);
#11376=ORIENTED_EDGE('',*,*,#8778,.F.);
#11377=ORIENTED_EDGE('',*,*,#8780,.F.);
#11378=ORIENTED_EDGE('',*,*,#8766,.F.);
#11379=ORIENTED_EDGE('',*,*,#8769,.F.);
#11380=ORIENTED_EDGE('',*,*,#8771,.F.);
#11381=ORIENTED_EDGE('',*,*,#8773,.F.);
#11382=ORIENTED_EDGE('',*,*,#8775,.F.);
#11383=ORIENTED_EDGE('',*,*,#8777,.F.);
#11384=ORIENTED_EDGE('',*,*,#8779,.F.);
#11385=ORIENTED_EDGE('',*,*,#8640,.F.);
#11386=ORIENTED_EDGE('',*,*,#8781,.T.);
#11387=ORIENTED_EDGE('',*,*,#8782,.T.);
#11388=ORIENTED_EDGE('',*,*,#8783,.F.);
#11389=ORIENTED_EDGE('',*,*,#8655,.F.);
#11390=ORIENTED_EDGE('',*,*,#8784,.T.);
#11391=ORIENTED_EDGE('',*,*,#8785,.T.);
#11392=ORIENTED_EDGE('',*,*,#8781,.F.);
#11393=ORIENTED_EDGE('',*,*,#8654,.F.);
#11394=ORIENTED_EDGE('',*,*,#8786,.T.);
#11395=ORIENTED_EDGE('',*,*,#8787,.T.);
#11396=ORIENTED_EDGE('',*,*,#8784,.F.);
#11397=ORIENTED_EDGE('',*,*,#8653,.F.);
#11398=ORIENTED_EDGE('',*,*,#8788,.T.);
#11399=ORIENTED_EDGE('',*,*,#8789,.T.);
#11400=ORIENTED_EDGE('',*,*,#8786,.F.);
#11401=ORIENTED_EDGE('',*,*,#8652,.F.);
#11402=ORIENTED_EDGE('',*,*,#8790,.T.);
#11403=ORIENTED_EDGE('',*,*,#8791,.T.);
#11404=ORIENTED_EDGE('',*,*,#8788,.F.);
#11405=ORIENTED_EDGE('',*,*,#8651,.F.);
#11406=ORIENTED_EDGE('',*,*,#8792,.T.);
#11407=ORIENTED_EDGE('',*,*,#8793,.T.);
#11408=ORIENTED_EDGE('',*,*,#8790,.F.);
#11409=ORIENTED_EDGE('',*,*,#8650,.F.);
#11410=ORIENTED_EDGE('',*,*,#8794,.T.);
#11411=ORIENTED_EDGE('',*,*,#8795,.T.);
#11412=ORIENTED_EDGE('',*,*,#8792,.F.);
#11413=ORIENTED_EDGE('',*,*,#8649,.F.);
#11414=ORIENTED_EDGE('',*,*,#8796,.T.);
#11415=ORIENTED_EDGE('',*,*,#8797,.T.);
#11416=ORIENTED_EDGE('',*,*,#8794,.F.);
#11417=ORIENTED_EDGE('',*,*,#8648,.F.);
#11418=ORIENTED_EDGE('',*,*,#8798,.T.);
#11419=ORIENTED_EDGE('',*,*,#8799,.T.);
#11420=ORIENTED_EDGE('',*,*,#8796,.F.);
#11421=ORIENTED_EDGE('',*,*,#8647,.F.);
#11422=ORIENTED_EDGE('',*,*,#8800,.T.);
#11423=ORIENTED_EDGE('',*,*,#8801,.T.);
#11424=ORIENTED_EDGE('',*,*,#8798,.F.);
#11425=ORIENTED_EDGE('',*,*,#8646,.F.);
#11426=ORIENTED_EDGE('',*,*,#8802,.T.);
#11427=ORIENTED_EDGE('',*,*,#8803,.T.);
#11428=ORIENTED_EDGE('',*,*,#8800,.F.);
#11429=ORIENTED_EDGE('',*,*,#8645,.F.);
#11430=ORIENTED_EDGE('',*,*,#8804,.T.);
#11431=ORIENTED_EDGE('',*,*,#8805,.T.);
#11432=ORIENTED_EDGE('',*,*,#8802,.F.);
#11433=ORIENTED_EDGE('',*,*,#8644,.F.);
#11434=ORIENTED_EDGE('',*,*,#8806,.T.);
#11435=ORIENTED_EDGE('',*,*,#8807,.T.);
#11436=ORIENTED_EDGE('',*,*,#8804,.F.);
#11437=ORIENTED_EDGE('',*,*,#8643,.F.);
#11438=ORIENTED_EDGE('',*,*,#8808,.T.);
#11439=ORIENTED_EDGE('',*,*,#8809,.T.);
#11440=ORIENTED_EDGE('',*,*,#8806,.F.);
#11441=ORIENTED_EDGE('',*,*,#8642,.F.);
#11442=ORIENTED_EDGE('',*,*,#8810,.T.);
#11443=ORIENTED_EDGE('',*,*,#8811,.T.);
#11444=ORIENTED_EDGE('',*,*,#8808,.F.);
#11445=ORIENTED_EDGE('',*,*,#8641,.F.);
#11446=ORIENTED_EDGE('',*,*,#8783,.T.);
#11447=ORIENTED_EDGE('',*,*,#8812,.T.);
#11448=ORIENTED_EDGE('',*,*,#8810,.F.);
#11449=ORIENTED_EDGE('',*,*,#8812,.F.);
#11450=ORIENTED_EDGE('',*,*,#8782,.F.);
#11451=ORIENTED_EDGE('',*,*,#8785,.F.);
#11452=ORIENTED_EDGE('',*,*,#8787,.F.);
#11453=ORIENTED_EDGE('',*,*,#8789,.F.);
#11454=ORIENTED_EDGE('',*,*,#8791,.F.);
#11455=ORIENTED_EDGE('',*,*,#8793,.F.);
#11456=ORIENTED_EDGE('',*,*,#8795,.F.);
#11457=ORIENTED_EDGE('',*,*,#8797,.F.);
#11458=ORIENTED_EDGE('',*,*,#8799,.F.);
#11459=ORIENTED_EDGE('',*,*,#8801,.F.);
#11460=ORIENTED_EDGE('',*,*,#8803,.F.);
#11461=ORIENTED_EDGE('',*,*,#8805,.F.);
#11462=ORIENTED_EDGE('',*,*,#8807,.F.);
#11463=ORIENTED_EDGE('',*,*,#8809,.F.);
#11464=ORIENTED_EDGE('',*,*,#8811,.F.);
#11465=ORIENTED_EDGE('',*,*,#8656,.F.);
#11466=ORIENTED_EDGE('',*,*,#8813,.T.);
#11467=ORIENTED_EDGE('',*,*,#8814,.T.);
#11468=ORIENTED_EDGE('',*,*,#8815,.F.);
#11469=ORIENTED_EDGE('',*,*,#8665,.F.);
#11470=ORIENTED_EDGE('',*,*,#8816,.T.);
#11471=ORIENTED_EDGE('',*,*,#8817,.T.);
#11472=ORIENTED_EDGE('',*,*,#8813,.F.);
#11473=ORIENTED_EDGE('',*,*,#8664,.F.);
#11474=ORIENTED_EDGE('',*,*,#8818,.T.);
#11475=ORIENTED_EDGE('',*,*,#8819,.T.);
#11476=ORIENTED_EDGE('',*,*,#8816,.F.);
#11477=ORIENTED_EDGE('',*,*,#8663,.F.);
#11478=ORIENTED_EDGE('',*,*,#8820,.T.);
#11479=ORIENTED_EDGE('',*,*,#8821,.T.);
#11480=ORIENTED_EDGE('',*,*,#8818,.F.);
#11481=ORIENTED_EDGE('',*,*,#8662,.F.);
#11482=ORIENTED_EDGE('',*,*,#8822,.T.);
#11483=ORIENTED_EDGE('',*,*,#8823,.T.);
#11484=ORIENTED_EDGE('',*,*,#8820,.F.);
#11485=ORIENTED_EDGE('',*,*,#8661,.F.);
#11486=ORIENTED_EDGE('',*,*,#8824,.T.);
#11487=ORIENTED_EDGE('',*,*,#8825,.T.);
#11488=ORIENTED_EDGE('',*,*,#8822,.F.);
#11489=ORIENTED_EDGE('',*,*,#8660,.F.);
#11490=ORIENTED_EDGE('',*,*,#8826,.T.);
#11491=ORIENTED_EDGE('',*,*,#8827,.T.);
#11492=ORIENTED_EDGE('',*,*,#8824,.F.);
#11493=ORIENTED_EDGE('',*,*,#8659,.F.);
#11494=ORIENTED_EDGE('',*,*,#8828,.T.);
#11495=ORIENTED_EDGE('',*,*,#8829,.T.);
#11496=ORIENTED_EDGE('',*,*,#8826,.F.);
#11497=ORIENTED_EDGE('',*,*,#8658,.F.);
#11498=ORIENTED_EDGE('',*,*,#8830,.T.);
#11499=ORIENTED_EDGE('',*,*,#8831,.T.);
#11500=ORIENTED_EDGE('',*,*,#8828,.F.);
#11501=ORIENTED_EDGE('',*,*,#8657,.F.);
#11502=ORIENTED_EDGE('',*,*,#8815,.T.);
#11503=ORIENTED_EDGE('',*,*,#8832,.T.);
#11504=ORIENTED_EDGE('',*,*,#8830,.F.);
#11505=ORIENTED_EDGE('',*,*,#8832,.F.);
#11506=ORIENTED_EDGE('',*,*,#8814,.F.);
#11507=ORIENTED_EDGE('',*,*,#8817,.F.);
#11508=ORIENTED_EDGE('',*,*,#8819,.F.);
#11509=ORIENTED_EDGE('',*,*,#8821,.F.);
#11510=ORIENTED_EDGE('',*,*,#8823,.F.);
#11511=ORIENTED_EDGE('',*,*,#8825,.F.);
#11512=ORIENTED_EDGE('',*,*,#8827,.F.);
#11513=ORIENTED_EDGE('',*,*,#8829,.F.);
#11514=ORIENTED_EDGE('',*,*,#8831,.F.);
#11515=ORIENTED_EDGE('',*,*,#8740,.F.);
#11516=ORIENTED_EDGE('',*,*,#8833,.T.);
#11517=ORIENTED_EDGE('',*,*,#8834,.T.);
#11518=ORIENTED_EDGE('',*,*,#8833,.F.);
#11519=ORIENTED_EDGE('',*,*,#8834,.F.);
#11520=ORIENTED_EDGE('',*,*,#8835,.F.);
#11521=ORIENTED_EDGE('',*,*,#8836,.T.);
#11522=ORIENTED_EDGE('',*,*,#8709,.F.);
#11523=ORIENTED_EDGE('',*,*,#8836,.F.);
#11524=ORIENTED_EDGE('',*,*,#8470,.F.);
#11525=ORIENTED_EDGE('',*,*,#8837,.T.);
#11526=ORIENTED_EDGE('',*,*,#8835,.T.);
#11527=ORIENTED_EDGE('',*,*,#8837,.F.);
#11528=ORIENTED_EDGE('',*,*,#8534,.F.);
#11529=ORIENTED_EDGE('',*,*,#8548,.F.);
#11530=ORIENTED_EDGE('',*,*,#8603,.F.);
#11531=ORIENTED_EDGE('',*,*,#8595,.F.);
#11532=ORIENTED_EDGE('',*,*,#8586,.F.);
#11533=ORIENTED_EDGE('',*,*,#8578,.F.);
#11534=ORIENTED_EDGE('',*,*,#8718,.T.);
#11535=ORIENTED_EDGE('',*,*,#8737,.F.);
#11536=ORIENTED_EDGE('',*,*,#8736,.F.);
#11537=ORIENTED_EDGE('',*,*,#8724,.F.);
#11538=ORIENTED_EDGE('',*,*,#8725,.F.);
#11539=ORIENTED_EDGE('',*,*,#8671,.F.);
#11540=ORIENTED_EDGE('',*,*,#8617,.F.);
#11541=ORIENTED_EDGE('',*,*,#8540,.F.);
#11542=ORIENTED_EDGE('',*,*,#8530,.F.);
#11543=ORIENTED_EDGE('',*,*,#8576,.F.);
#11544=ORIENTED_EDGE('',*,*,#8719,.T.);
#11545=ORIENTED_EDGE('',*,*,#8579,.F.);
#11546=ORIENTED_EDGE('',*,*,#8688,.F.);
#11547=ORIENTED_EDGE('',*,*,#8716,.T.);
#11548=ORIENTED_EDGE('',*,*,#8698,.F.);
#11549=ORIENTED_EDGE('',*,*,#8693,.F.);
#15478=CONICAL_SURFACE('',#16760,15.45,0.785398163397451);
#15479=CONICAL_SURFACE('',#16768,15.45,0.785398163397451);
#15480=CONICAL_SURFACE('',#16895,26.5,0.785398163397451);
#15481=CONICAL_SURFACE('',#16963,21.525,0.759762754875774);
#15543=ADVANCED_FACE('',(#1815),#15478,.F.);
#15544=ADVANCED_FACE('',(#1816),#1563,.F.);
#15545=ADVANCED_FACE('',(#1817,#939),#1062,.F.);
#15546=ADVANCED_FACE('',(#1818),#15479,.F.);
#15547=ADVANCED_FACE('',(#1819,#940),#1063,.F.);
#15548=ADVANCED_FACE('',(#1820),#814,.T.);
#15549=ADVANCED_FACE('',(#1821),#815,.T.);
#15550=ADVANCED_FACE('',(#1822),#1064,.T.);
#15551=ADVANCED_FACE('',(#1823),#1065,.F.);
#15552=ADVANCED_FACE('',(#1824),#1564,.T.);
#15553=ADVANCED_FACE('',(#1825),#1066,.T.);
#15554=ADVANCED_FACE('',(#1826),#816,.T.);
#15555=ADVANCED_FACE('',(#1827),#817,.T.);
#15556=ADVANCED_FACE('',(#1828),#818,.T.);
#15557=ADVANCED_FACE('',(#1829),#819,.T.);
#15558=ADVANCED_FACE('',(#1830),#820,.T.);
#15559=ADVANCED_FACE('',(#1831),#1067,.T.);
#15560=ADVANCED_FACE('',(#1832),#821,.T.);
#15561=ADVANCED_FACE('',(#1833),#822,.T.);
#15562=ADVANCED_FACE('',(#1834),#823,.T.);
#15563=ADVANCED_FACE('',(#1835),#824,.T.);
#15564=ADVANCED_FACE('',(#1836),#825,.T.);
#15565=ADVANCED_FACE('',(#1837),#1565,.T.);
#15566=ADVANCED_FACE('',(#1838),#1068,.T.);
#15567=ADVANCED_FACE('',(#1839),#1566,.T.);
#15568=ADVANCED_FACE('',(#1840),#1069,.T.);
#15569=ADVANCED_FACE('',(#1841),#1567,.T.);
#15570=ADVANCED_FACE('',(#1842),#231,.T.);
#15571=ADVANCED_FACE('',(#1843),#232,.T.);
#15572=ADVANCED_FACE('',(#1844),#1568,.T.);
#15573=ADVANCED_FACE('',(#1845),#1569,.T.);
#15574=ADVANCED_FACE('',(#1846),#1070,.T.);
#15575=ADVANCED_FACE('',(#1847),#233,.T.);
#15576=ADVANCED_FACE('',(#1848),#1570,.T.);
#15577=ADVANCED_FACE('',(#1849),#1571,.T.);
#15578=ADVANCED_FACE('',(#1850),#234,.T.);
#15579=ADVANCED_FACE('',(#1851),#235,.T.);
#15580=ADVANCED_FACE('',(#1852),#1572,.T.);
#15581=ADVANCED_FACE('',(#1853),#1573,.T.);
#15582=ADVANCED_FACE('',(#1854),#236,.T.);
#15583=ADVANCED_FACE('',(#1855),#237,.T.);
#15584=ADVANCED_FACE('',(#1856),#1574,.T.);
#15585=ADVANCED_FACE('',(#1857),#1575,.T.);
#15586=ADVANCED_FACE('',(#1858),#238,.T.);
#15587=ADVANCED_FACE('',(#1859),#239,.T.);
#15588=ADVANCED_FACE('',(#1860),#1576,.T.);
#15589=ADVANCED_FACE('',(#1861),#1577,.T.);
#15590=ADVANCED_FACE('',(#1862),#240,.T.);
#15591=ADVANCED_FACE('',(#1863),#1578,.T.);
#15592=ADVANCED_FACE('',(#1864),#241,.T.);
#15593=ADVANCED_FACE('',(#1865),#1579,.T.);
#15594=ADVANCED_FACE('',(#1866),#1580,.T.);
#15595=ADVANCED_FACE('',(#1867),#242,.T.);
#15596=ADVANCED_FACE('',(#1868),#1581,.T.);
#15597=ADVANCED_FACE('',(#1869),#243,.T.);
#15598=ADVANCED_FACE('',(#1870,#941,#942,#943,#944),#1071,.T.);
#15599=ADVANCED_FACE('',(#1871),#1072,.T.);
#15600=ADVANCED_FACE('',(#1872),#1582,.T.);
#15601=ADVANCED_FACE('',(#1873),#1583,.T.);
#15602=ADVANCED_FACE('',(#1874),#1584,.T.);
#15603=ADVANCED_FACE('',(#1875),#1073,.T.);
#15604=ADVANCED_FACE('',(#1876),#1585,.T.);
#15605=ADVANCED_FACE('',(#1877),#1586,.T.);
#15606=ADVANCED_FACE('',(#1878),#1587,.T.);
#15607=ADVANCED_FACE('',(#1879),#1588,.T.);
#15608=ADVANCED_FACE('',(#1880),#1074,.T.);
#15609=ADVANCED_FACE('',(#1881),#1075,.T.);
#15610=ADVANCED_FACE('',(#1882),#1589,.T.);
#15611=ADVANCED_FACE('',(#1883),#1590,.T.);
#15612=ADVANCED_FACE('',(#1884),#1076,.F.);
#15613=ADVANCED_FACE('',(#1885),#244,.T.);
#15614=ADVANCED_FACE('',(#1886),#1591,.T.);
#15615=ADVANCED_FACE('',(#1887),#1592,.T.);
#15616=ADVANCED_FACE('',(#1888),#245,.T.);
#15617=ADVANCED_FACE('',(#1889),#1593,.T.);
#15618=ADVANCED_FACE('',(#1890),#1077,.T.);
#15619=ADVANCED_FACE('',(#1891),#1594,.T.);
#15620=ADVANCED_FACE('',(#1892),#1595,.T.);
#15621=ADVANCED_FACE('',(#1893),#1078,.T.);
#15622=ADVANCED_FACE('',(#1894),#215,.T.);
#15623=ADVANCED_FACE('',(#1895),#15480,.T.);
#15624=ADVANCED_FACE('',(#1896,#945),#1079,.T.);
#15625=ADVANCED_FACE('',(#1897),#216,.T.);
#15626=ADVANCED_FACE('',(#1898),#1596,.T.);
#15627=ADVANCED_FACE('',(#1899),#217,.T.);
#15628=ADVANCED_FACE('',(#1900),#1597,.T.);
#15629=ADVANCED_FACE('',(#1901),#218,.T.);
#15630=ADVANCED_FACE('',(#1902),#1598,.T.);
#15631=ADVANCED_FACE('',(#1903),#219,.T.);
#15632=ADVANCED_FACE('',(#1904),#1599,.T.);
#15633=ADVANCED_FACE('',(#1905),#220,.T.);
#15634=ADVANCED_FACE('',(#1906),#221,.T.);
#15635=ADVANCED_FACE('',(#1907),#222,.T.);
#15636=ADVANCED_FACE('',(#1908),#1600,.T.);
#15637=ADVANCED_FACE('',(#1909),#223,.T.);
#15638=ADVANCED_FACE('',(#1910,#946),#1080,.F.);
#15639=ADVANCED_FACE('',(#1911),#1601,.F.);
#15640=ADVANCED_FACE('',(#1912),#1081,.F.);
#15641=ADVANCED_FACE('',(#1913),#1602,.F.);
#15642=ADVANCED_FACE('',(#1914),#826,.F.);
#15643=ADVANCED_FACE('',(#1915),#827,.F.);
#15644=ADVANCED_FACE('',(#1916),#828,.F.);
#15645=ADVANCED_FACE('',(#1917),#829,.F.);
#15646=ADVANCED_FACE('',(#1918),#830,.F.);
#15647=ADVANCED_FACE('',(#1919),#831,.F.);
#15648=ADVANCED_FACE('',(#1920),#832,.F.);
#15649=ADVANCED_FACE('',(#1921),#833,.F.);
#15650=ADVANCED_FACE('',(#1922),#834,.F.);
#15651=ADVANCED_FACE('',(#1923),#835,.F.);
#15652=ADVANCED_FACE('',(#1924),#836,.F.);
#15653=ADVANCED_FACE('',(#1925),#1082,.T.);
#15654=ADVANCED_FACE('',(#1926),#1083,.F.);
#15655=ADVANCED_FACE('',(#1927),#1084,.F.);
#15656=ADVANCED_FACE('',(#1928),#1085,.F.);
#15657=ADVANCED_FACE('',(#1929),#1086,.F.);
#15658=ADVANCED_FACE('',(#1930),#1087,.F.);
#15659=ADVANCED_FACE('',(#1931),#1088,.F.);
#15660=ADVANCED_FACE('',(#1932),#1089,.F.);
#15661=ADVANCED_FACE('',(#1933),#1090,.F.);
#15662=ADVANCED_FACE('',(#1934),#1091,.F.);
#15663=ADVANCED_FACE('',(#1935),#837,.F.);
#15664=ADVANCED_FACE('',(#1936),#838,.F.);
#15665=ADVANCED_FACE('',(#1937),#839,.F.);
#15666=ADVANCED_FACE('',(#1938),#840,.F.);
#15667=ADVANCED_FACE('',(#1939),#841,.F.);
#15668=ADVANCED_FACE('',(#1940),#842,.F.);
#15669=ADVANCED_FACE('',(#1941),#843,.F.);
#15670=ADVANCED_FACE('',(#1942),#844,.F.);
#15671=ADVANCED_FACE('',(#1943),#845,.F.);
#15672=ADVANCED_FACE('',(#1944),#846,.F.);
#15673=ADVANCED_FACE('',(#1945),#847,.F.);
#15674=ADVANCED_FACE('',(#1946),#848,.F.);
#15675=ADVANCED_FACE('',(#1947),#849,.F.);
#15676=ADVANCED_FACE('',(#1948),#850,.F.);
#15677=ADVANCED_FACE('',(#1949),#851,.F.);
#15678=ADVANCED_FACE('',(#1950),#852,.F.);
#15679=ADVANCED_FACE('',(#1951),#1092,.T.);
#15680=ADVANCED_FACE('',(#1952),#1093,.F.);
#15681=ADVANCED_FACE('',(#1953),#1094,.F.);
#15682=ADVANCED_FACE('',(#1954),#1095,.F.);
#15683=ADVANCED_FACE('',(#1955),#1096,.F.);
#15684=ADVANCED_FACE('',(#1956),#1097,.F.);
#15685=ADVANCED_FACE('',(#1957),#1098,.F.);
#15686=ADVANCED_FACE('',(#1958),#1099,.F.);
#15687=ADVANCED_FACE('',(#1959),#1100,.F.);
#15688=ADVANCED_FACE('',(#1960),#1101,.F.);
#15689=ADVANCED_FACE('',(#1961),#1102,.F.);
#15690=ADVANCED_FACE('',(#1962),#1103,.F.);
#15691=ADVANCED_FACE('',(#1963),#1603,.F.);
#15692=ADVANCED_FACE('',(#1964),#1104,.T.);
#15693=ADVANCED_FACE('',(#1965),#15481,.F.);
#15694=ADVANCED_FACE('',(#1966),#1604,.F.);
#15695=ADVANCED_FACE('',(#1967),#1105,.T.);
#15696=ADVANCED_FACE('',(#1968),#1106,.T.);
#15697=ADVANCED_FACE('',(#1969),#1107,.T.);
#16517=CLOSED_SHELL('',(#15543,#15544,#15545,#15546,#15547,#15548,#15549,
#15550,#15551,#15552,#15553,#15554,#15555,#15556,#15557,#15558,#15559,#15560,
#15561,#15562,#15563,#15564,#15565,#15566,#15567,#15568,#15569,#15570,#15571,
#15572,#15573,#15574,#15575,#15576,#15577,#15578,#15579,#15580,#15581,#15582,
#15583,#15584,#15585,#15586,#15587,#15588,#15589,#15590,#15591,#15592,#15593,
#15594,#15595,#15596,#15597,#15598,#15599,#15600,#15601,#15602,#15603,#15604,
#15605,#15606,#15607,#15608,#15609,#15610,#15611,#15612,#15613,#15614,#15615,
#15616,#15617,#15618,#15619,#15620,#15621,#15622,#15623,#15624,#15625,#15626,
#15627,#15628,#15629,#15630,#15631,#15632,#15633,#15634,#15635,#15636,#15637,
#15638,#15639,#15640,#15641,#15642,#15643,#15644,#15645,#15646,#15647,#15648,
#15649,#15650,#15651,#15652,#15653,#15654,#15655,#15656,#15657,#15658,#15659,
#15660,#15661,#15662,#15663,#15664,#15665,#15666,#15667,#15668,#15669,#15670,
#15671,#15672,#15673,#15674,#15675,#15676,#15677,#15678,#15679,#15680,#15681,
#15682,#15683,#15684,#15685,#15686,#15687,#15688,#15689,#15690,#15691,#15692,
#15693,#15694,#15695,#15696,#15697));
#16759=AXIS2_PLACEMENT_3D('',#22165,#18125,#18126);
#16760=AXIS2_PLACEMENT_3D('',#22166,#18127,#18128);
#16761=AXIS2_PLACEMENT_3D('',#22169,#18129,#18130);
#16762=AXIS2_PLACEMENT_3D('',#22170,#18131,#18132);
#16763=AXIS2_PLACEMENT_3D('',#22173,#18134,#18135);
#16764=AXIS2_PLACEMENT_3D('',#22174,#18136,#18137);
#16765=AXIS2_PLACEMENT_3D('',#22176,#18138,#18139);
#16766=AXIS2_PLACEMENT_3D('',#22178,#18141,#18142);
#16767=AXIS2_PLACEMENT_3D('',#22180,#18143,#18144);
#16768=AXIS2_PLACEMENT_3D('',#22181,#18145,#18146);
#16769=AXIS2_PLACEMENT_3D('',#22183,#18147,#18148);
#16770=AXIS2_PLACEMENT_3D('',#22185,#18150,#18151);
#16771=AXIS2_PLACEMENT_3D('',#22188,#18152,#18153);
#16772=AXIS2_PLACEMENT_3D('',#22196,#18157,#18158);
#16773=AXIS2_PLACEMENT_3D('',#22202,#18161,#18162);
#16774=AXIS2_PLACEMENT_3D('',#22382,#18167,#18168);
#16775=AXIS2_PLACEMENT_3D('',#22385,#18169,#18170);
#16776=AXIS2_PLACEMENT_3D('',#22388,#18173,#18174);
#16777=AXIS2_PLACEMENT_3D('',#22404,#18182,#18183);
#16778=AXIS2_PLACEMENT_3D('',#22408,#18185,#18186);
#16779=AXIS2_PLACEMENT_3D('',#22414,#18190,#18191);
#16780=AXIS2_PLACEMENT_3D('',#22417,#18193,#18194);
#16781=AXIS2_PLACEMENT_3D('',#22418,#18195,#18196);
#16782=AXIS2_PLACEMENT_3D('',#22420,#18197,#18198);
#16783=AXIS2_PLACEMENT_3D('',#22793,#18207,#18208);
#16784=AXIS2_PLACEMENT_3D('',#22931,#18216,#18217);
#16785=AXIS2_PLACEMENT_3D('',#22935,#18219,#18220);
#16786=AXIS2_PLACEMENT_3D('',#22937,#18222,#18223);
#16787=AXIS2_PLACEMENT_3D('',#22943,#18227,#18228);
#16788=AXIS2_PLACEMENT_3D('',#22946,#18230,#18231);
#16789=AXIS2_PLACEMENT_3D('',#22947,#18232,#18233);
#16790=AXIS2_PLACEMENT_3D('',#22951,#18236,#18237);
#16791=AXIS2_PLACEMENT_3D('',#22954,#18238,#18239);
#16792=AXIS2_PLACEMENT_3D('',#22958,#18241,#18242);
#16793=AXIS2_PLACEMENT_3D('',#22960,#18244,#18245);
#16794=AXIS2_PLACEMENT_3D('',#22962,#18246,#18247);
#16795=AXIS2_PLACEMENT_3D('',#22963,#18248,#18249);
#16796=AXIS2_PLACEMENT_3D('',#22964,#18250,#18251);
#16797=AXIS2_PLACEMENT_3D('',#22965,#18252,#18253);
#16798=AXIS2_PLACEMENT_3D('',#22966,#18254,#18255);
#16799=AXIS2_PLACEMENT_3D('',#22967,#18256,#18257);
#16800=AXIS2_PLACEMENT_3D('',#22984,#18260,#18261);
#16801=AXIS2_PLACEMENT_3D('',#22999,#18264,#18265);
#16802=AXIS2_PLACEMENT_3D('',#23003,#18268,#18269);
#16803=AXIS2_PLACEMENT_3D('',#23005,#18270,#18271);
#16804=AXIS2_PLACEMENT_3D('',#23007,#18272,#18273);
#16805=AXIS2_PLACEMENT_3D('',#23008,#18274,#18275);
#16806=AXIS2_PLACEMENT_3D('',#23009,#18276,#18277);
#16807=AXIS2_PLACEMENT_3D('',#23020,#18279,#18280);
#16808=AXIS2_PLACEMENT_3D('',#23037,#18283,#18284);
#16809=AXIS2_PLACEMENT_3D('',#23040,#18285,#18286);
#16810=AXIS2_PLACEMENT_3D('',#23041,#18287,#18288);
#16811=AXIS2_PLACEMENT_3D('',#23042,#18289,#18290);
#16812=AXIS2_PLACEMENT_3D('',#23043,#18291,#18292);
#16813=AXIS2_PLACEMENT_3D('',#23045,#18293,#18294);
#16814=AXIS2_PLACEMENT_3D('',#23046,#18295,#18296);
#16815=AXIS2_PLACEMENT_3D('',#23047,#18297,#18298);
#16816=AXIS2_PLACEMENT_3D('',#23049,#18300,#18301);
#16817=AXIS2_PLACEMENT_3D('',#23051,#18303,#18304);
#16818=AXIS2_PLACEMENT_3D('',#23054,#18305,#18306);
#16819=AXIS2_PLACEMENT_3D('',#23056,#18307,#18308);
#16820=AXIS2_PLACEMENT_3D('',#23057,#18309,#18310);
#16821=AXIS2_PLACEMENT_3D('',#23058,#18311,#18312);
#16822=AXIS2_PLACEMENT_3D('',#23061,#18313,#18314);
#16823=AXIS2_PLACEMENT_3D('',#23062,#18315,#18316);
#16824=AXIS2_PLACEMENT_3D('',#23063,#18317,#18318);
#16825=AXIS2_PLACEMENT_3D('',#23064,#18319,#18320);
#16826=AXIS2_PLACEMENT_3D('',#23067,#18323,#18324);
#16827=AXIS2_PLACEMENT_3D('',#23070,#18327,#18328);
#16828=AXIS2_PLACEMENT_3D('',#23072,#18329,#18330);
#16829=AXIS2_PLACEMENT_3D('',#23073,#18331,#18332);
#16830=AXIS2_PLACEMENT_3D('',#23074,#18333,#18334);
#16831=AXIS2_PLACEMENT_3D('',#23076,#18335,#18336);
#16832=AXIS2_PLACEMENT_3D('',#23077,#18337,#18338);
#16833=AXIS2_PLACEMENT_3D('',#23078,#18339,#18340);
#16834=AXIS2_PLACEMENT_3D('',#23079,#18341,#18342);
#16835=AXIS2_PLACEMENT_3D('',#23081,#18344,#18345);
#16836=AXIS2_PLACEMENT_3D('',#23084,#18348,#18349);
#16837=AXIS2_PLACEMENT_3D('',#23086,#18350,#18351);
#16838=AXIS2_PLACEMENT_3D('',#23087,#18352,#18353);
#16839=AXIS2_PLACEMENT_3D('',#23088,#18354,#18355);
#16840=AXIS2_PLACEMENT_3D('',#23089,#18356,#18357);
#16841=AXIS2_PLACEMENT_3D('',#23091,#18358,#18359);
#16842=AXIS2_PLACEMENT_3D('',#23093,#18361,#18362);
#16843=AXIS2_PLACEMENT_3D('',#23095,#18363,#18364);
#16844=AXIS2_PLACEMENT_3D('',#23096,#18365,#18366);
#16845=AXIS2_PLACEMENT_3D('',#23097,#18367,#18368);
#16846=AXIS2_PLACEMENT_3D('',#23098,#18369,#18370);
#16847=AXIS2_PLACEMENT_3D('',#23099,#18371,#18372);
#16848=AXIS2_PLACEMENT_3D('',#23101,#18374,#18375);
#16849=AXIS2_PLACEMENT_3D('',#23104,#18376,#18377);
#16850=AXIS2_PLACEMENT_3D('',#23106,#18378,#18379);
#16851=AXIS2_PLACEMENT_3D('',#23107,#18380,#18381);
#16852=AXIS2_PLACEMENT_3D('',#23108,#18382,#18383);
#16853=AXIS2_PLACEMENT_3D('',#23111,#18386,#18387);
#16854=AXIS2_PLACEMENT_3D('',#23112,#18388,#18389);
#16855=AXIS2_PLACEMENT_3D('',#23113,#18390,#18391);
#16856=AXIS2_PLACEMENT_3D('',#23259,#18411,#18412);
#16857=AXIS2_PLACEMENT_3D('',#23261,#18414,#18415);
#16858=AXIS2_PLACEMENT_3D('',#23262,#18416,#18417);
#16859=AXIS2_PLACEMENT_3D('',#23263,#18418,#18419);
#16860=AXIS2_PLACEMENT_3D('',#23266,#18421,#18422);
#16861=AXIS2_PLACEMENT_3D('',#23267,#18423,#18424);
#16862=AXIS2_PLACEMENT_3D('',#23269,#18426,#18427);
#16863=AXIS2_PLACEMENT_3D('',#23271,#18429,#18430);
#16864=AXIS2_PLACEMENT_3D('',#23275,#18432,#18433);
#16865=AXIS2_PLACEMENT_3D('',#23277,#18435,#18436);
#16866=AXIS2_PLACEMENT_3D('',#23278,#18437,#18438);
#16867=AXIS2_PLACEMENT_3D('',#23293,#18440,#18441);
#16868=AXIS2_PLACEMENT_3D('',#23294,#18442,#18443);
#16869=AXIS2_PLACEMENT_3D('',#23295,#18444,#18445);
#16870=AXIS2_PLACEMENT_3D('',#23296,#18446,#18447);
#16871=AXIS2_PLACEMENT_3D('',#23297,#18448,#18449);
#16872=AXIS2_PLACEMENT_3D('',#23314,#18451,#18452);
#16873=AXIS2_PLACEMENT_3D('',#23329,#18453,#18454);
#16874=AXIS2_PLACEMENT_3D('',#23331,#18456,#18457);
#16875=AXIS2_PLACEMENT_3D('',#23334,#18458,#18459);
#16876=AXIS2_PLACEMENT_3D('',#23335,#18460,#18461);
#16877=AXIS2_PLACEMENT_3D('',#23336,#18462,#18463);
#16878=AXIS2_PLACEMENT_3D('',#23337,#18464,#18465);
#16879=AXIS2_PLACEMENT_3D('',#23354,#18467,#18468);
#16880=AXIS2_PLACEMENT_3D('',#23371,#18470,#18471);
#16881=AXIS2_PLACEMENT_3D('',#23374,#18472,#18473);
#16882=AXIS2_PLACEMENT_3D('',#23376,#18474,#18475);
#16883=AXIS2_PLACEMENT_3D('',#23377,#18476,#18477);
#16884=AXIS2_PLACEMENT_3D('',#23378,#18478,#18479);
#16885=AXIS2_PLACEMENT_3D('',#23381,#18482,#18483);
#16886=AXIS2_PLACEMENT_3D('',#23385,#18486,#18487);
#16887=AXIS2_PLACEMENT_3D('',#23398,#18489,#18490);
#16888=AXIS2_PLACEMENT_3D('',#23415,#18493,#18494);
#16889=AXIS2_PLACEMENT_3D('',#23416,#18495,#18496);
#16890=AXIS2_PLACEMENT_3D('',#23417,#18497,#18498);
#16891=AXIS2_PLACEMENT_3D('',#23419,#18499,#18500);
#16892=AXIS2_PLACEMENT_3D('',#23421,#18501,#18502);
#16893=AXIS2_PLACEMENT_3D('',#23423,#18503,#18504);
#16894=AXIS2_PLACEMENT_3D('',#23424,#18505,#18506);
#16895=AXIS2_PLACEMENT_3D('',#23425,#18507,#18508);
#16896=AXIS2_PLACEMENT_3D('',#23429,#18510,#18511);
#16897=AXIS2_PLACEMENT_3D('',#23430,#18512,#18513);
#16898=AXIS2_PLACEMENT_3D('',#23431,#18514,#18515);
#16899=AXIS2_PLACEMENT_3D('',#23433,#18516,#18517);
#16900=AXIS2_PLACEMENT_3D('',#23434,#18518,#18519);
#16901=AXIS2_PLACEMENT_3D('',#23436,#18520,#18521);
#16902=AXIS2_PLACEMENT_3D('',#23438,#18522,#18523);
#16903=AXIS2_PLACEMENT_3D('',#23439,#18524,#18525);
#16904=AXIS2_PLACEMENT_3D('',#23440,#18526,#18527);
#16905=AXIS2_PLACEMENT_3D('',#23443,#18529,#18530);
#16906=AXIS2_PLACEMENT_3D('',#23444,#18531,#18532);
#16907=AXIS2_PLACEMENT_3D('',#23447,#18534,#18535);
#16908=AXIS2_PLACEMENT_3D('',#23449,#18537,#18538);
#16909=AXIS2_PLACEMENT_3D('',#23450,#18539,#18540);
#16910=AXIS2_PLACEMENT_3D('',#23451,#18541,#18542);
#16911=AXIS2_PLACEMENT_3D('',#23452,#18543,#18544);
#16912=AXIS2_PLACEMENT_3D('',#23455,#18545,#18546);
#16913=AXIS2_PLACEMENT_3D('',#23459,#18548,#18549);
#16914=AXIS2_PLACEMENT_3D('',#23461,#18551,#18552);
#16915=AXIS2_PLACEMENT_3D('',#23462,#18553,#18554);
#16916=AXIS2_PLACEMENT_3D('',#23463,#18555,#18556);
#16917=AXIS2_PLACEMENT_3D('',#23464,#18557,#18558);
#16918=AXIS2_PLACEMENT_3D('',#23466,#18559,#18560);
#16919=AXIS2_PLACEMENT_3D('',#23469,#18562,#18563);
#16920=AXIS2_PLACEMENT_3D('',#23470,#18564,#18565);
#16921=AXIS2_PLACEMENT_3D('',#23471,#18566,#18567);
#16922=AXIS2_PLACEMENT_3D('',#23472,#18568,#18569);
#16923=AXIS2_PLACEMENT_3D('',#23473,#18570,#18571);
#16924=AXIS2_PLACEMENT_3D('',#23488,#18572,#18573);
#16925=AXIS2_PLACEMENT_3D('',#23489,#18574,#18575);
#16926=AXIS2_PLACEMENT_3D('',#23490,#18576,#18577);
#16927=AXIS2_PLACEMENT_3D('',#23491,#18578,#18579);
#16928=AXIS2_PLACEMENT_3D('',#23493,#18580,#18581);
#16929=AXIS2_PLACEMENT_3D('',#23494,#18582,#18583);
#16930=AXIS2_PLACEMENT_3D('',#23495,#18584,#18585);
#16931=AXIS2_PLACEMENT_3D('',#23496,#18586,#18587);
#16932=AXIS2_PLACEMENT_3D('',#23512,#18589,#18590);
#16933=AXIS2_PLACEMENT_3D('',#23513,#18591,#18592);
#16934=AXIS2_PLACEMENT_3D('',#23516,#18594,#18595);
#16935=AXIS2_PLACEMENT_3D('',#23517,#18596,#18597);
#16936=AXIS2_PLACEMENT_3D('',#23519,#18599,#18600);
#16937=AXIS2_PLACEMENT_3D('',#23521,#18602,#18603);
#16938=AXIS2_PLACEMENT_3D('',#23643,#18615,#18616);
#16939=AXIS2_PLACEMENT_3D('',#23644,#18617,#18618);
#16940=AXIS2_PLACEMENT_3D('',#23650,#18622,#18623);
#16941=AXIS2_PLACEMENT_3D('',#23654,#18626,#18627);
#16942=AXIS2_PLACEMENT_3D('',#23658,#18630,#18631);
#16943=AXIS2_PLACEMENT_3D('',#23662,#18634,#18635);
#16944=AXIS2_PLACEMENT_3D('',#23666,#18638,#18639);
#16945=AXIS2_PLACEMENT_3D('',#23670,#18642,#18643);
#16946=AXIS2_PLACEMENT_3D('',#23674,#18646,#18647);
#16947=AXIS2_PLACEMENT_3D('',#23676,#18649,#18650);
#16948=AXIS2_PLACEMENT_3D('',#23853,#18667,#18668);
#16949=AXIS2_PLACEMENT_3D('',#23854,#18669,#18670);
#16950=AXIS2_PLACEMENT_3D('',#23860,#18674,#18675);
#16951=AXIS2_PLACEMENT_3D('',#23864,#18678,#18679);
#16952=AXIS2_PLACEMENT_3D('',#23868,#18682,#18683);
#16953=AXIS2_PLACEMENT_3D('',#23872,#18686,#18687);
#16954=AXIS2_PLACEMENT_3D('',#23876,#18690,#18691);
#16955=AXIS2_PLACEMENT_3D('',#23880,#18694,#18695);
#16956=AXIS2_PLACEMENT_3D('',#23884,#18698,#18699);
#16957=AXIS2_PLACEMENT_3D('',#23888,#18702,#18703);
#16958=AXIS2_PLACEMENT_3D('',#23892,#18706,#18707);
#16959=AXIS2_PLACEMENT_3D('',#23894,#18709,#18710);
#16960=AXIS2_PLACEMENT_3D('',#23895,#18711,#18712);
#16961=AXIS2_PLACEMENT_3D('',#23898,#18714,#18715);
#16962=AXIS2_PLACEMENT_3D('',#23899,#18716,#18717);
#16963=AXIS2_PLACEMENT_3D('',#23900,#18718,#18719);
#16964=AXIS2_PLACEMENT_3D('',#23902,#18720,#18721);
#16965=AXIS2_PLACEMENT_3D('',#23904,#18723,#18724);
#16966=AXIS2_PLACEMENT_3D('',#23906,#18726,#18727);
#16967=AXIS2_PLACEMENT_3D('',#23907,#18728,#18729);
#16968=AXIS2_PLACEMENT_3D('',#23908,#18730,#18731);
#18125=DIRECTION('axis',(0.,0.,1.));
#18126=DIRECTION('refdir',(1.,0.,0.));
#18127=DIRECTION('center_axis',(1.,0.,0.));
#18128=DIRECTION('ref_axis',(0.,-1.,0.));
#18129=DIRECTION('center_axis',(-1.,0.,0.));
#18130=DIRECTION('ref_axis',(0.,-1.,0.));
#18131=DIRECTION('center_axis',(-1.,0.,0.));
#18132=DIRECTION('ref_axis',(0.,-1.,0.));
#18133=DIRECTION('',(0.707106781186546,0.707106781186549,-8.65956056235495E-17));
#18134=DIRECTION('center_axis',(1.,0.,0.));
#18135=DIRECTION('ref_axis',(0.,-1.,0.));
#18136=DIRECTION('center_axis',(1.,0.,0.));
#18137=DIRECTION('ref_axis',(0.,1.,0.));
#18138=DIRECTION('center_axis',(1.,0.,0.));
#18139=DIRECTION('ref_axis',(0.,1.,0.));
#18140=DIRECTION('',(1.,0.,0.));
#18141=DIRECTION('center_axis',(-1.,0.,0.));
#18142=DIRECTION('ref_axis',(0.,0.,1.));
#18143=DIRECTION('center_axis',(1.,0.,0.));
#18144=DIRECTION('ref_axis',(0.,0.,-1.));
#18145=DIRECTION('center_axis',(-1.,0.,0.));
#18146=DIRECTION('ref_axis',(0.,1.,0.));
#18147=DIRECTION('center_axis',(-1.,0.,0.));
#18148=DIRECTION('ref_axis',(0.,1.,0.));
#18149=DIRECTION('',(0.707106781186546,0.707106781186549,-8.65956056235495E-17));
#18150=DIRECTION('center_axis',(1.,0.,0.));
#18151=DIRECTION('ref_axis',(0.,0.,-1.));
#18152=DIRECTION('center_axis',(1.,0.,0.));
#18153=DIRECTION('ref_axis',(0.,-1.,1.83697019872103E-16));
#18154=DIRECTION('',(0.,0.,-1.));
#18155=DIRECTION('',(0.,-1.,0.));
#18156=DIRECTION('',(0.,0.,1.));
#18157=DIRECTION('center_axis',(1.,0.,0.));
#18158=DIRECTION('ref_axis',(0.,1.,-6.12323399573677E-17));
#18159=DIRECTION('',(0.,0.,1.));
#18160=DIRECTION('',(0.,1.,0.));
#18161=DIRECTION('center_axis',(1.,0.,0.));
#18162=DIRECTION('ref_axis',(0.,-2.44929359829471E-16,-1.));
#18163=DIRECTION('',(0.,1.,0.));
#18164=DIRECTION('',(0.,0.,-1.));
#18165=DIRECTION('',(0.457581580857944,0.,-0.889167642719608));
#18166=DIRECTION('',(-0.457581580857943,0.,0.889167642719609));
#18167=DIRECTION('center_axis',(0.889167642719609,0.,0.457581580857943));
#18168=DIRECTION('ref_axis',(0.457581580857943,0.,-0.889167642719609));
#18169=DIRECTION('center_axis',(0.889167642719609,0.,0.457581580857943));
#18170=DIRECTION('ref_axis',(-0.457581580857943,0.,0.889167642719609));
#18171=DIRECTION('',(0.,-1.,0.));
#18172=DIRECTION('',(0.,1.,0.));
#18173=DIRECTION('center_axis',(0.,1.,0.));
#18174=DIRECTION('ref_axis',(1.,0.,0.));
#18175=DIRECTION('',(0.813733471206735,0.,-0.581238193719096));
#18176=DIRECTION('',(1.,0.,0.));
#18177=DIRECTION('',(0.707106781186547,0.,0.707106781186548));
#18178=DIRECTION('',(0.,0.,1.));
#18179=DIRECTION('',(-0.707106781186548,0.,0.707106781186547));
#18180=DIRECTION('',(-1.,0.,0.));
#18181=DIRECTION('',(0.,0.,-1.));
#18182=DIRECTION('center_axis',(0.,-1.,0.));
#18183=DIRECTION('ref_axis',(-0.707106781186548,0.,0.707106781186548));
#18184=DIRECTION('',(-1.,0.,0.));
#18185=DIRECTION('center_axis',(0.,-1.,0.));
#18186=DIRECTION('ref_axis',(0.707106781186548,0.,0.707106781186547));
#18187=DIRECTION('',(0.,0.,1.));
#18188=DIRECTION('',(1.,0.,0.));
#18189=DIRECTION('',(0.,0.,-1.));
#18190=DIRECTION('center_axis',(-0.813733471206735,0.,0.581238193719096));
#18191=DIRECTION('ref_axis',(0.410997468263393,-0.707106781186548,0.575396455568749));
#18192=DIRECTION('',(-0.813733471206735,0.,0.581238193719096));
#18193=DIRECTION('center_axis',(-0.813733471206735,0.,0.581238193719096));
#18194=DIRECTION('ref_axis',(0.410997468263392,-0.707106781186551,0.575396455568747));
#18195=DIRECTION('center_axis',(0.581238193719096,0.,0.813733471206735));
#18196=DIRECTION('ref_axis',(0.813733471206735,0.,-0.581238193719096));
#18197=DIRECTION('center_axis',(-0.581238193719096,0.,-0.813733471206735));
#18198=DIRECTION('ref_axis',(-0.813733471206735,0.,0.581238193719096));
#18199=DIRECTION('',(0.,-1.,0.));
#18200=DIRECTION('',(0.813733471206735,0.,-0.581238193719096));
#18201=DIRECTION('',(0.,1.,0.));
#18202=DIRECTION('',(-0.707106781186548,-0.707106781186548,0.));
#18203=DIRECTION('',(0.,0.707106781186546,0.707106781186549));
#18204=DIRECTION('',(1.08368419587492E-12,-0.707106781186914,-0.707106781186181));
#18205=DIRECTION('',(-0.392473756018299,-0.725569174564963,-0.565255450002923));
#18206=DIRECTION('',(0.0228311464870028,0.69541471336182,0.718245859848831));
#18207=DIRECTION('center_axis',(-0.500000000000002,0.707106781186544,-0.500000000000003));
#18208=DIRECTION('ref_axis',(-0.707106781186548,0.,0.707106781186547));
#18209=DIRECTION('',(0.499999999999997,0.707106781186549,0.500000000000002));
#18210=DIRECTION('',(0.707106781186548,0.,-0.707106781186547));
#18211=DIRECTION('',(-0.499999999999998,-0.707106781186551,-0.499999999999997));
#18212=DIRECTION('',(-0.707106781186548,0.,0.707106781186547));
#18213=DIRECTION('',(0.565255450002919,0.725569174564966,0.392473756018301));
#18214=DIRECTION('',(-0.718245859848833,-0.695414713361818,-0.022831146487005));
#18215=DIRECTION('',(0.707106781186178,0.707106781186917,-1.08089518879373E-12));
#18216=DIRECTION('center_axis',(0.,0.,1.));
#18217=DIRECTION('ref_axis',(-0.707106781186546,0.707106781186549,0.));
#18218=DIRECTION('',(0.,0.,1.));
#18219=DIRECTION('center_axis',(0.,0.,1.));
#18220=DIRECTION('ref_axis',(-1.,0.,0.));
#18221=DIRECTION('',(0.,0.,-1.));
#18222=DIRECTION('center_axis',(-1.,0.,0.));
#18223=DIRECTION('ref_axis',(0.,0.,1.));
#18224=DIRECTION('',(0.,1.,0.));
#18225=DIRECTION('',(0.,0.,-1.));
#18226=DIRECTION('',(0.,-1.,0.));
#18227=DIRECTION('center_axis',(0.,1.,0.));
#18228=DIRECTION('ref_axis',(-0.923879532511287,0.,-0.382683432365089));
#18229=DIRECTION('',(0.,-1.,0.));
#18230=DIRECTION('center_axis',(0.,1.,0.));
#18231=DIRECTION('ref_axis',(-0.707106781186548,0.,-0.707106781186547));
#18232=DIRECTION('center_axis',(-0.707106781186547,0.,-0.707106781186548));
#18233=DIRECTION('ref_axis',(-0.707106781186548,0.,0.707106781186547));
#18234=DIRECTION('',(0.,1.,0.));
#18235=DIRECTION('',(0.707106781186548,0.,-0.707106781186547));
#18236=DIRECTION('center_axis',(1.,0.,0.));
#18237=DIRECTION('ref_axis',(0.,-0.70710678118655,-0.707106781186545));
#18238=DIRECTION('center_axis',(1.,0.,0.));
#18239=DIRECTION('ref_axis',(0.,-1.,-2.96059473233374E-15));
#18240=DIRECTION('',(1.,0.,0.));
#18241=DIRECTION('center_axis',(-1.,0.,0.));
#18242=DIRECTION('ref_axis',(0.,0.,-1.));
#18243=DIRECTION('',(-1.,0.,0.));
#18244=DIRECTION('center_axis',(-0.816496580927727,-0.408248290463863,-0.408248290463861));
#18245=DIRECTION('ref_axis',(0.577350269189624,-0.577350269189629,-0.577350269189624));
#18246=DIRECTION('center_axis',(0.,-1.,0.));
#18247=DIRECTION('ref_axis',(0.70710678118655,0.,-0.707106781186545));
#18248=DIRECTION('center_axis',(0.,0.,-1.));
#18249=DIRECTION('ref_axis',(0.707106781186546,-0.707106781186549,0.));
#18250=DIRECTION('center_axis',(0.40824829046386,-0.816496580927727,0.408248290463865));
#18251=DIRECTION('ref_axis',(-0.577350269189623,-0.577350269189626,-0.577350269189628));
#18252=DIRECTION('center_axis',(0.,0.,-1.));
#18253=DIRECTION('ref_axis',(-0.707106781186546,-0.707106781186549,0.));
#18254=DIRECTION('center_axis',(0.,-1.,0.));
#18255=DIRECTION('ref_axis',(-0.707106781186546,0.,-0.707106781186549));
#18256=DIRECTION('center_axis',(0.,0.,1.));
#18257=DIRECTION('ref_axis',(0.707106781186548,-0.707106781186548,0.));
#18258=DIRECTION('',(0.,0.,1.));
#18259=DIRECTION('',(0.,0.,-1.));
#18260=DIRECTION('center_axis',(0.,1.,0.));
#18261=DIRECTION('ref_axis',(0.70710678118655,0.,-0.707106781186545));
#18262=DIRECTION('',(0.,1.,0.));
#18263=DIRECTION('',(0.,-1.,0.));
#18264=DIRECTION('center_axis',(0.,0.,-1.));
#18265=DIRECTION('ref_axis',(-1.,0.,0.));
#18266=DIRECTION('',(0.,-1.,0.));
#18267=DIRECTION('',(1.,0.,0.));
#18268=DIRECTION('center_axis',(0.,0.,1.));
#18269=DIRECTION('ref_axis',(1.,0.,0.));
#18270=DIRECTION('center_axis',(0.813733471206734,-1.72081073455594E-15,
-0.581238193719098));
#18271=DIRECTION('ref_axis',(0.581238193719098,0.,0.813733471206734));
#18272=DIRECTION('center_axis',(0.,1.,0.));
#18273=DIRECTION('ref_axis',(1.,0.,0.));
#18274=DIRECTION('center_axis',(0.,0.,1.));
#18275=DIRECTION('ref_axis',(0.,1.,0.));
#18276=DIRECTION('center_axis',(0.,1.,0.));
#18277=DIRECTION('ref_axis',(0.889167642719608,0.,0.457581580857944));
#18278=DIRECTION('',(0.,1.,0.));
#18279=DIRECTION('center_axis',(0.,0.,-1.));
#18280=DIRECTION('ref_axis',(0.707106781186543,0.707106781186552,0.));
#18281=DIRECTION('',(0.,0.,1.));
#18282=DIRECTION('',(0.,0.,-1.));
#18283=DIRECTION('center_axis',(0.141866792680437,-0.885380737596912,0.442690368798457));
#18284=DIRECTION('ref_axis',(0.27019821896378,0.464866593220407,0.843144099769698));
#18285=DIRECTION('center_axis',(1.,0.,0.));
#18286=DIRECTION('ref_axis',(0.,0.,1.));
#18287=DIRECTION('center_axis',(0.,1.,0.));
#18288=DIRECTION('ref_axis',(0.581238193719098,0.,0.813733471206734));
#18289=DIRECTION('center_axis',(-0.813733471206734,0.,0.581238193719098));
#18290=DIRECTION('ref_axis',(0.,1.,0.));
#18291=DIRECTION('center_axis',(-0.141866792680436,-0.885380737596912,-0.442690368798456));
#18292=DIRECTION('ref_axis',(0.27019821896378,-0.464866593220407,0.843144099769698));
#18293=DIRECTION('center_axis',(0.,-1.,0.));
#18294=DIRECTION('ref_axis',(0.581238193719094,0.,0.813733471206737));
#18295=DIRECTION('center_axis',(1.,0.,0.));
#18296=DIRECTION('ref_axis',(0.,-0.707106781186549,0.707106781186546));
#18297=DIRECTION('center_axis',(0.,1.,0.));
#18298=DIRECTION('ref_axis',(0.305177431007984,0.,0.952295508549404));
#18299=DIRECTION('',(0.,-1.,0.));
#18300=DIRECTION('center_axis',(0.813733471206735,0.,-0.581238193719096));
#18301=DIRECTION('ref_axis',(0.410997468263393,0.707106781186548,0.575396455568749));
#18302=DIRECTION('',(-0.813733471206735,0.,0.581238193719096));
#18303=DIRECTION('center_axis',(-0.182143211721526,-0.879465224064609,0.439732612032305));
#18304=DIRECTION('ref_axis',(-0.336556770590777,0.475963149477969,0.812519920068745));
#18305=DIRECTION('center_axis',(0.707106781186549,1.57009245868377E-15,
0.707106781186546));
#18306=DIRECTION('ref_axis',(-0.707106781186546,0.,0.707106781186549));
#18307=DIRECTION('center_axis',(0.,1.,0.));
#18308=DIRECTION('ref_axis',(0.,0.,1.));
#18309=DIRECTION('center_axis',(-1.,0.,1.48029736616687E-15));
#18310=DIRECTION('ref_axis',(0.,1.,0.));
#18311=DIRECTION('center_axis',(0.182143211721527,-0.879465224064609,-0.439732612032306));
#18312=DIRECTION('ref_axis',(-0.336556770590777,-0.475963149477967,0.812519920068746));
#18313=DIRECTION('center_axis',(0.,-1.,0.));
#18314=DIRECTION('ref_axis',(0.,0.,1.));
#18315=DIRECTION('center_axis',(0.707106781186547,0.,0.707106781186548));
#18316=DIRECTION('ref_axis',(-0.5,-0.707106781186548,0.5));
#18317=DIRECTION('center_axis',(-1.,0.,0.));
#18318=DIRECTION('ref_axis',(0.,-0.707106781186549,0.707106781186546));
#18319=DIRECTION('center_axis',(0.,1.,0.));
#18320=DIRECTION('ref_axis',(-0.382683432365088,0.,0.923879532511287));
#18321=DIRECTION('',(0.,1.,0.));
#18322=DIRECTION('',(0.,-1.,0.));
#18323=DIRECTION('center_axis',(1.,0.,0.));
#18324=DIRECTION('ref_axis',(0.,0.707106781186548,0.707106781186548));
#18325=DIRECTION('',(-1.,0.,0.));
#18326=DIRECTION('',(1.,0.,0.));
#18327=DIRECTION('center_axis',(0.,0.,1.));
#18328=DIRECTION('ref_axis',(1.,0.,0.));
#18329=DIRECTION('center_axis',(0.,1.,0.));
#18330=DIRECTION('ref_axis',(-0.707106781186548,0.,0.707106781186547));
#18331=DIRECTION('center_axis',(-0.707106781186548,0.,-0.707106781186548));
#18332=DIRECTION('ref_axis',(0.,1.,0.));
#18333=DIRECTION('center_axis',(0.,0.,1.));
#18334=DIRECTION('ref_axis',(1.,0.,0.));
#18335=DIRECTION('center_axis',(0.,-1.,0.));
#18336=DIRECTION('ref_axis',(-0.707106781186547,0.,0.707106781186548));
#18337=DIRECTION('center_axis',(0.,0.,1.));
#18338=DIRECTION('ref_axis',(-0.707106781186546,-0.707106781186549,0.));
#18339=DIRECTION('center_axis',(-0.707106781186547,0.,-0.707106781186548));
#18340=DIRECTION('ref_axis',(-0.499999999999999,-0.707106781186549,0.499999999999998));
#18341=DIRECTION('center_axis',(0.,1.,0.));
#18342=DIRECTION('ref_axis',(-0.923879532511287,0.,0.382683432365089));
#18343=DIRECTION('',(0.,1.,0.));
#18344=DIRECTION('center_axis',(0.707106781186547,0.,0.707106781186548));
#18345=DIRECTION('ref_axis',(-0.500000000000001,0.707106781186548,0.499999999999998));
#18346=DIRECTION('',(-0.707106781186547,0.,-0.707106781186548));
#18347=DIRECTION('',(0.707106781186547,0.,0.707106781186548));
#18348=DIRECTION('center_axis',(0.182143211721528,-0.879465224064609,0.439732612032306));
#18349=DIRECTION('ref_axis',(-0.336556770590778,-0.475963149477968,-0.812519920068745));
#18350=DIRECTION('center_axis',(0.,-1.,0.));
#18351=DIRECTION('ref_axis',(0.,0.,-1.));
#18352=DIRECTION('center_axis',(-1.,0.,0.));
#18353=DIRECTION('ref_axis',(0.,-1.,0.));
#18354=DIRECTION('center_axis',(0.707106781186548,5.23364152894591E-16,
-0.707106781186547));
#18355=DIRECTION('ref_axis',(-0.707106781186547,0.,-0.707106781186548));
#18356=DIRECTION('center_axis',(1.,0.,0.));
#18357=DIRECTION('ref_axis',(0.,-0.70710678118655,-0.707106781186545));
#18358=DIRECTION('center_axis',(-1.,-2.96059473233374E-15,-2.96059473233375E-15));
#18359=DIRECTION('ref_axis',(2.96059473233375E-15,0.,-1.));
#18360=DIRECTION('',(1.,0.,0.));
#18361=DIRECTION('center_axis',(-0.816496580927726,-0.408248290463864,-0.408248290463862));
#18362=DIRECTION('ref_axis',(0.577350269189625,-0.577350269189627,-0.577350269189625));
#18363=DIRECTION('center_axis',(0.,-1.,0.));
#18364=DIRECTION('ref_axis',(0.707106781186549,0.,-0.707106781186546));
#18365=DIRECTION('center_axis',(0.,0.,-1.));
#18366=DIRECTION('ref_axis',(0.707106781186546,-0.707106781186549,0.));
#18367=DIRECTION('center_axis',(0.707106781186548,0.,-0.707106781186547));
#18368=DIRECTION('ref_axis',(-0.500000000000001,-0.707106781186548,-0.499999999999998));
#18369=DIRECTION('center_axis',(0.707106781186548,0.,-0.707106781186547));
#18370=DIRECTION('ref_axis',(0.,-1.,0.));
#18371=DIRECTION('center_axis',(0.,1.,0.));
#18372=DIRECTION('ref_axis',(-0.38268343236509,0.,-0.923879532511287));
#18373=DIRECTION('',(0.,-1.,0.));
#18374=DIRECTION('center_axis',(-0.816496580927726,0.408248290463864,-0.408248290463862));
#18375=DIRECTION('ref_axis',(0.577350269189625,0.577350269189627,-0.577350269189625));
#18376=DIRECTION('center_axis',(1.,0.,0.));
#18377=DIRECTION('ref_axis',(0.,0.,-1.));
#18378=DIRECTION('center_axis',(0.,0.,-1.));
#18379=DIRECTION('ref_axis',(0.707106781186546,0.707106781186549,0.));
#18380=DIRECTION('center_axis',(0.,1.,0.));
#18381=DIRECTION('ref_axis',(0.707106781186549,0.,-0.707106781186546));
#18382=DIRECTION('center_axis',(-1.,0.,0.));
#18383=DIRECTION('ref_axis',(0.,0.70710678118655,-0.707106781186545));
#18384=DIRECTION('',(1.,0.,0.));
#18385=DIRECTION('',(-1.,0.,0.));
#18386=DIRECTION('center_axis',(0.,0.,1.));
#18387=DIRECTION('ref_axis',(1.,0.,0.));
#18388=DIRECTION('center_axis',(0.,0.,-1.));
#18389=DIRECTION('ref_axis',(-0.707106781186546,-0.707106781186549,0.));
#18390=DIRECTION('center_axis',(0.,0.,1.));
#18391=DIRECTION('ref_axis',(1.,0.,0.));
#18392=DIRECTION('',(-1.,0.,0.));
#18393=DIRECTION('',(-1.,0.,0.));
#18394=DIRECTION('',(0.,-1.,0.));
#18395=DIRECTION('',(-1.,0.,0.));
#18396=DIRECTION('',(0.,1.,0.));
#18397=DIRECTION('',(-1.,0.,0.));
#18398=DIRECTION('',(0.,1.,0.));
#18399=DIRECTION('',(1.,0.,0.));
#18400=DIRECTION('',(0.,-1.,0.));
#18401=DIRECTION('',(-0.555699076657711,0.831383507294779,0.));
#18402=DIRECTION('',(0.,-1.,0.));
#18403=DIRECTION('',(-1.,0.,0.));
#18404=DIRECTION('',(0.,1.,0.));
#18405=DIRECTION('',(1.,0.,0.));
#18406=DIRECTION('',(0.556032582744129,-0.831160494084562,0.));
#18407=DIRECTION('',(0.,1.,0.));
#18408=DIRECTION('',(1.,0.,0.));
#18409=DIRECTION('',(0.,-1.,0.));
#18410=DIRECTION('',(-1.,0.,0.));
#18411=DIRECTION('center_axis',(-0.707106781186548,0.,0.707106781186547));
#18412=DIRECTION('ref_axis',(0.707106781186547,0.,0.707106781186548));
#18413=DIRECTION('',(-0.707106781186547,0.,-0.707106781186548));
#18414=DIRECTION('center_axis',(-0.707106781186547,0.,-0.707106781186548));
#18415=DIRECTION('ref_axis',(-0.500000000000001,-0.707106781186548,0.499999999999998));
#18416=DIRECTION('center_axis',(0.,0.,-1.));
#18417=DIRECTION('ref_axis',(-0.707106781186546,-0.707106781186549,0.));
#18418=DIRECTION('center_axis',(0.,0.,1.));
#18419=DIRECTION('ref_axis',(0.707106781186546,-0.707106781186549,0.));
#18420=DIRECTION('',(0.,0.,1.));
#18421=DIRECTION('center_axis',(0.,0.,1.));
#18422=DIRECTION('ref_axis',(0.,-1.,0.));
#18423=DIRECTION('center_axis',(0.,0.,-1.));
#18424=DIRECTION('ref_axis',(-1.,0.,0.));
#18425=DIRECTION('',(0.,1.,0.));
#18426=DIRECTION('center_axis',(0.,-1.,0.));
#18427=DIRECTION('ref_axis',(0.707106781186548,0.,-0.707106781186547));
#18428=DIRECTION('',(0.,-1.,0.));
#18429=DIRECTION('center_axis',(0.,0.,-1.));
#18430=DIRECTION('ref_axis',(0.707106781186546,0.707106781186549,0.));
#18431=DIRECTION('',(0.,0.,1.));
#18432=DIRECTION('center_axis',(0.,0.,1.));
#18433=DIRECTION('ref_axis',(1.,0.,0.));
#18434=DIRECTION('',(0.,0.,-1.));
#18435=DIRECTION('center_axis',(-1.,0.,0.));
#18436=DIRECTION('ref_axis',(0.,-0.707106781186548,0.707106781186548));
#18437=DIRECTION('center_axis',(0.,0.,1.));
#18438=DIRECTION('ref_axis',(0.707106781186543,-0.707106781186552,0.));
#18439=DIRECTION('',(0.,0.,1.));
#18440=DIRECTION('center_axis',(1.,0.,0.));
#18441=DIRECTION('ref_axis',(0.,0.,-1.));
#18442=DIRECTION('center_axis',(-1.,0.,0.));
#18443=DIRECTION('ref_axis',(0.,1.,0.));
#18444=DIRECTION('center_axis',(1.,0.,0.));
#18445=DIRECTION('ref_axis',(0.,0.,-1.));
#18446=DIRECTION('center_axis',(-1.,0.,0.));
#18447=DIRECTION('ref_axis',(0.,1.,0.));
#18448=DIRECTION('center_axis',(0.,0.,-1.));
#18449=DIRECTION('ref_axis',(-0.707106781186548,-0.707106781186548,0.));
#18450=DIRECTION('',(0.,0.,1.));
#18451=DIRECTION('center_axis',(0.,1.,0.));
#18452=DIRECTION('ref_axis',(-0.707106781186548,0.,-0.707106781186548));
#18453=DIRECTION('center_axis',(0.,1.,0.));
#18454=DIRECTION('ref_axis',(1.,0.,0.));
#18455=DIRECTION('',(-1.,0.,0.));
#18456=DIRECTION('center_axis',(-0.408248290463863,-0.816496580927726,-0.408248290463863));
#18457=DIRECTION('ref_axis',(-0.577350269189626,0.577350269189626,-0.577350269189626));
#18458=DIRECTION('center_axis',(-1.,0.,0.));
#18459=DIRECTION('ref_axis',(0.,0.,-1.));
#18460=DIRECTION('center_axis',(0.,1.,0.));
#18461=DIRECTION('ref_axis',(-1.,0.,0.));
#18462=DIRECTION('center_axis',(-5.92118946466749E-15,0.,-1.));
#18463=DIRECTION('ref_axis',(0.,1.,0.));
#18464=DIRECTION('center_axis',(0.,1.,0.));
#18465=DIRECTION('ref_axis',(-0.707106781186548,0.,-0.707106781186548));
#18466=DIRECTION('',(0.,-1.,0.));
#18467=DIRECTION('center_axis',(0.,0.,1.));
#18468=DIRECTION('ref_axis',(-0.707106781186548,0.707106781186548,0.));
#18469=DIRECTION('',(0.,0.,-1.));
#18470=DIRECTION('center_axis',(-0.816496580927726,0.408248290463865,-0.408248290463861));
#18471=DIRECTION('ref_axis',(0.577350269189631,0.577350269189626,-0.577350269189621));
#18472=DIRECTION('center_axis',(1.,0.,0.));
#18473=DIRECTION('ref_axis',(0.,0.,-1.));
#18474=DIRECTION('center_axis',(0.,0.,-1.));
#18475=DIRECTION('ref_axis',(0.707106781186546,0.707106781186549,0.));
#18476=DIRECTION('center_axis',(0.,1.,0.));
#18477=DIRECTION('ref_axis',(0.70710678118655,0.,-0.707106781186545));
#18478=DIRECTION('center_axis',(-1.,0.,0.));
#18479=DIRECTION('ref_axis',(0.,0.70710678118655,-0.707106781186545));
#18480=DIRECTION('',(-1.,0.,0.));
#18481=DIRECTION('',(1.,0.,0.));
#18482=DIRECTION('center_axis',(0.,0.,-1.));
#18483=DIRECTION('ref_axis',(-1.,0.,0.));
#18484=DIRECTION('',(0.,1.,0.));
#18485=DIRECTION('',(-1.,0.,0.));
#18486=DIRECTION('center_axis',(0.,1.,0.));
#18487=DIRECTION('ref_axis',(0.70710678118655,0.,-0.707106781186545));
#18488=DIRECTION('',(0.,-1.,0.));
#18489=DIRECTION('center_axis',(0.,0.,-1.));
#18490=DIRECTION('ref_axis',(0.707106781186548,0.707106781186548,0.));
#18491=DIRECTION('',(0.,0.,1.));
#18492=DIRECTION('',(0.,0.,-1.));
#18493=DIRECTION('center_axis',(1.,0.,0.));
#18494=DIRECTION('ref_axis',(0.,0.,-1.));
#18495=DIRECTION('center_axis',(-1.,0.,0.));
#18496=DIRECTION('ref_axis',(0.,1.,0.));
#18497=DIRECTION('center_axis',(1.,0.,0.));
#18498=DIRECTION('ref_axis',(0.,0.,-1.));
#18499=DIRECTION('center_axis',(-1.,0.,0.));
#18500=DIRECTION('ref_axis',(0.,-1.,1.83697019872103E-16));
#18501=DIRECTION('center_axis',(0.,-1.,-1.22464679914735E-16));
#18502=DIRECTION('ref_axis',(0.,-1.22464679914735E-16,1.));
#18503=DIRECTION('center_axis',(1.,0.,0.));
#18504=DIRECTION('ref_axis',(0.,-1.,3.06161699786838E-17));
#18505=DIRECTION('center_axis',(1.,0.,0.));
#18506=DIRECTION('ref_axis',(0.,-1.,3.06161699786838E-17));
#18507=DIRECTION('center_axis',(-1.,0.,0.));
#18508=DIRECTION('ref_axis',(0.,1.,0.));
#18509=DIRECTION('',(-0.707106781186546,-0.707106781186549,-8.65956056235495E-17));
#18510=DIRECTION('center_axis',(-1.,0.,0.));
#18511=DIRECTION('ref_axis',(0.,-1.,3.06161699786838E-17));
#18512=DIRECTION('center_axis',(-1.,0.,0.));
#18513=DIRECTION('ref_axis',(0.,-1.,3.06161699786838E-17));
#18514=DIRECTION('center_axis',(1.,0.,0.));
#18515=DIRECTION('ref_axis',(0.,0.,-1.));
#18516=DIRECTION('center_axis',(-1.,0.,0.));
#18517=DIRECTION('ref_axis',(0.,1.,0.));
#18518=DIRECTION('center_axis',(1.,0.,0.));
#18519=DIRECTION('ref_axis',(0.,0.,-1.));
#18520=DIRECTION('center_axis',(0.,-1.,-1.22464679914735E-16));
#18521=DIRECTION('ref_axis',(0.,-1.22464679914735E-16,1.));
#18522=DIRECTION('center_axis',(1.,0.,0.));
#18523=DIRECTION('ref_axis',(0.,-1.,1.83697019872103E-16));
#18524=DIRECTION('center_axis',(1.,0.,0.));
#18525=DIRECTION('ref_axis',(0.,-1.,1.83697019872103E-16));
#18526=DIRECTION('center_axis',(1.,0.,0.));
#18527=DIRECTION('ref_axis',(0.,1.,0.));
#18528=DIRECTION('',(-1.,0.,0.));
#18529=DIRECTION('center_axis',(-1.,0.,0.));
#18530=DIRECTION('ref_axis',(0.,-1.,1.83697019872103E-16));
#18531=DIRECTION('center_axis',(-1.,0.,0.));
#18532=DIRECTION('ref_axis',(0.,-2.44929359829471E-16,-1.));
#18533=DIRECTION('',(1.,0.,0.));
#18534=DIRECTION('center_axis',(-1.,0.,0.));
#18535=DIRECTION('ref_axis',(0.,1.,-6.12323399573677E-17));
#18536=DIRECTION('',(-1.,0.,0.));
#18537=DIRECTION('center_axis',(-1.,0.,0.));
#18538=DIRECTION('ref_axis',(0.,1.,0.));
#18539=DIRECTION('center_axis',(-1.,0.,0.));
#18540=DIRECTION('ref_axis',(0.,-1.,1.83697019872103E-16));
#18541=DIRECTION('center_axis',(1.,0.,0.));
#18542=DIRECTION('ref_axis',(0.,0.,-1.));
#18543=DIRECTION('center_axis',(-1.,0.,0.));
#18544=DIRECTION('ref_axis',(0.,0.707106781186548,-0.707106781186548));
#18545=DIRECTION('center_axis',(-1.,0.,0.));
#18546=DIRECTION('ref_axis',(0.,1.,0.));
#18547=DIRECTION('',(-1.,0.,0.));
#18548=DIRECTION('center_axis',(1.,0.,0.));
#18549=DIRECTION('ref_axis',(0.,0.,-1.));
#18550=DIRECTION('',(1.,0.,0.));
#18551=DIRECTION('center_axis',(0.,1.,0.));
#18552=DIRECTION('ref_axis',(0.,0.,1.));
#18553=DIRECTION('center_axis',(0.,1.,0.));
#18554=DIRECTION('ref_axis',(-0.707106781186548,0.,0.707106781186548));
#18555=DIRECTION('center_axis',(0.,-1.,0.));
#18556=DIRECTION('ref_axis',(-0.707106781186547,0.,0.707106781186547));
#18557=DIRECTION('center_axis',(1.,0.,0.));
#18558=DIRECTION('ref_axis',(0.,-0.707106781186548,-0.707106781186548));
#18559=DIRECTION('center_axis',(1.,0.,0.));
#18560=DIRECTION('ref_axis',(0.,-1.,0.));
#18561=DIRECTION('',(1.,0.,0.));
#18562=DIRECTION('center_axis',(-1.,0.,0.));
#18563=DIRECTION('ref_axis',(0.,0.,-1.));
#18564=DIRECTION('center_axis',(0.,-1.,0.));
#18565=DIRECTION('ref_axis',(0.,0.,-1.));
#18566=DIRECTION('center_axis',(1.48029736616687E-15,0.,1.));
#18567=DIRECTION('ref_axis',(-1.,0.,1.48029736616687E-15));
#18568=DIRECTION('center_axis',(0.,1.,0.));
#18569=DIRECTION('ref_axis',(0.707106781186548,0.,0.707106781186547));
#18570=DIRECTION('center_axis',(0.,0.,-1.));
#18571=DIRECTION('ref_axis',(-0.707106781186548,-0.707106781186548,0.));
#18572=DIRECTION('center_axis',(0.,-1.,0.));
#18573=DIRECTION('ref_axis',(0.,0.,-1.));
#18574=DIRECTION('center_axis',(0.,1.,0.));
#18575=DIRECTION('ref_axis',(-0.707106781186547,0.,0.707106781186547));
#18576=DIRECTION('center_axis',(1.,0.,0.));
#18577=DIRECTION('ref_axis',(0.,0.,-1.));
#18578=DIRECTION('center_axis',(0.,1.,0.));
#18579=DIRECTION('ref_axis',(0.,0.,1.));
#18580=DIRECTION('center_axis',(1.48029736616687E-15,0.,1.));
#18581=DIRECTION('ref_axis',(0.,1.,0.));
#18582=DIRECTION('center_axis',(0.,-1.,0.));
#18583=DIRECTION('ref_axis',(0.707106781186548,0.,0.707106781186547));
#18584=DIRECTION('center_axis',(0.,1.,0.));
#18585=DIRECTION('ref_axis',(0.707106781186548,0.,0.707106781186547));
#18586=DIRECTION('center_axis',(0.,0.,1.));
#18587=DIRECTION('ref_axis',(-0.707106781186548,0.707106781186548,0.));
#18588=DIRECTION('',(0.,0.,-1.));
#18589=DIRECTION('center_axis',(1.,0.,0.));
#18590=DIRECTION('ref_axis',(0.,0.,-1.));
#18591=DIRECTION('center_axis',(-1.,0.,0.));
#18592=DIRECTION('ref_axis',(0.,0.,1.));
#18593=DIRECTION('',(0.,1.,0.));
#18594=DIRECTION('center_axis',(-1.,0.,0.));
#18595=DIRECTION('ref_axis',(0.,0.,-1.));
#18596=DIRECTION('center_axis',(0.,1.,0.));
#18597=DIRECTION('ref_axis',(-0.707106781186548,0.,0.707106781186547));
#18598=DIRECTION('',(0.,-1.,0.));
#18599=DIRECTION('center_axis',(0.,0.,1.));
#18600=DIRECTION('ref_axis',(1.,0.,0.));
#18601=DIRECTION('',(0.,1.,0.));
#18602=DIRECTION('center_axis',(0.,1.,0.));
#18603=DIRECTION('ref_axis',(0.707106781186546,0.,0.707106781186549));
#18604=DIRECTION('',(0.,0.,-1.));
#18605=DIRECTION('',(0.,0.,-1.));
#18606=DIRECTION('',(0.,0.,-1.));
#18607=DIRECTION('',(0.,0.,-1.));
#18608=DIRECTION('',(0.,0.,-1.));
#18609=DIRECTION('',(0.,0.,-1.));
#18610=DIRECTION('',(0.,0.,-1.));
#18611=DIRECTION('',(0.,0.,-1.));
#18612=DIRECTION('',(0.,0.,-1.));
#18613=DIRECTION('',(0.,0.,-1.));
#18614=DIRECTION('',(0.,0.,-1.));
#18615=DIRECTION('center_axis',(0.,0.,1.));
#18616=DIRECTION('ref_axis',(1.,0.,0.));
#18617=DIRECTION('center_axis',(0.,-1.,0.));
#18618=DIRECTION('ref_axis',(-1.,0.,0.));
#18619=DIRECTION('',(0.,0.,-1.));
#18620=DIRECTION('',(-1.,0.,0.));
#18621=DIRECTION('',(0.,0.,-1.));
#18622=DIRECTION('center_axis',(1.,0.,0.));
#18623=DIRECTION('ref_axis',(0.,-1.,0.));
#18624=DIRECTION('',(0.,0.,-1.));
#18625=DIRECTION('',(0.,-1.,0.));
#18626=DIRECTION('center_axis',(0.,1.,0.));
#18627=DIRECTION('ref_axis',(1.,0.,0.));
#18628=DIRECTION('',(0.,0.,-1.));
#18629=DIRECTION('',(1.,0.,0.));
#18630=DIRECTION('center_axis',(-1.,0.,0.));
#18631=DIRECTION('ref_axis',(0.,1.,0.));
#18632=DIRECTION('',(0.,0.,-1.));
#18633=DIRECTION('',(0.,1.,0.));
#18634=DIRECTION('center_axis',(0.,-1.,0.));
#18635=DIRECTION('ref_axis',(-1.,0.,0.));
#18636=DIRECTION('',(0.,0.,-1.));
#18637=DIRECTION('',(-1.,0.,0.));
#18638=DIRECTION('center_axis',(-1.,0.,0.));
#18639=DIRECTION('ref_axis',(0.,1.,0.));
#18640=DIRECTION('',(0.,0.,-1.));
#18641=DIRECTION('',(0.,1.,0.));
#18642=DIRECTION('center_axis',(0.,-1.,0.));
#18643=DIRECTION('ref_axis',(-1.,0.,0.));
#18644=DIRECTION('',(0.,0.,-1.));
#18645=DIRECTION('',(-1.,0.,0.));
#18646=DIRECTION('center_axis',(1.,0.,0.));
#18647=DIRECTION('ref_axis',(0.,-1.,0.));
#18648=DIRECTION('',(0.,-1.,0.));
#18649=DIRECTION('center_axis',(0.,0.,-1.));
#18650=DIRECTION('ref_axis',(-1.,0.,0.));
#18651=DIRECTION('',(0.,0.,-1.));
#18652=DIRECTION('',(0.,0.,-1.));
#18653=DIRECTION('',(0.,0.,-1.));
#18654=DIRECTION('',(0.,0.,-1.));
#18655=DIRECTION('',(0.,0.,-1.));
#18656=DIRECTION('',(0.,0.,-1.));
#18657=DIRECTION('',(0.,0.,-1.));
#18658=DIRECTION('',(0.,0.,-1.));
#18659=DIRECTION('',(0.,0.,-1.));
#18660=DIRECTION('',(0.,0.,-1.));
#18661=DIRECTION('',(0.,0.,-1.));
#18662=DIRECTION('',(0.,0.,-1.));
#18663=DIRECTION('',(0.,0.,-1.));
#18664=DIRECTION('',(0.,0.,-1.));
#18665=DIRECTION('',(0.,0.,-1.));
#18666=DIRECTION('',(0.,0.,-1.));
#18667=DIRECTION('center_axis',(0.,0.,1.));
#18668=DIRECTION('ref_axis',(1.,0.,0.));
#18669=DIRECTION('center_axis',(-0.831383507294779,-0.555699076657711,0.));
#18670=DIRECTION('ref_axis',(-0.555699076657711,0.831383507294779,0.));
#18671=DIRECTION('',(0.,0.,-1.));
#18672=DIRECTION('',(-0.555699076657711,0.831383507294779,0.));
#18673=DIRECTION('',(0.,0.,-1.));
#18674=DIRECTION('center_axis',(0.,-1.,0.));
#18675=DIRECTION('ref_axis',(-1.,0.,0.));
#18676=DIRECTION('',(0.,0.,-1.));
#18677=DIRECTION('',(-1.,0.,0.));
#18678=DIRECTION('center_axis',(1.,0.,0.));
#18679=DIRECTION('ref_axis',(0.,-1.,0.));
#18680=DIRECTION('',(0.,0.,-1.));
#18681=DIRECTION('',(0.,-1.,0.));
#18682=DIRECTION('center_axis',(0.,1.,0.));
#18683=DIRECTION('ref_axis',(1.,0.,0.));
#18684=DIRECTION('',(0.,0.,-1.));
#18685=DIRECTION('',(1.,0.,0.));
#18686=DIRECTION('center_axis',(-1.,0.,0.));
#18687=DIRECTION('ref_axis',(0.,1.,0.));
#18688=DIRECTION('',(0.,0.,-1.));
#18689=DIRECTION('',(0.,1.,0.));
#18690=DIRECTION('center_axis',(0.831160494084562,0.556032582744129,0.));
#18691=DIRECTION('ref_axis',(0.556032582744129,-0.831160494084562,0.));
#18692=DIRECTION('',(0.,0.,-1.));
#18693=DIRECTION('',(0.556032582744129,-0.831160494084562,0.));
#18694=DIRECTION('center_axis',(0.,1.,0.));
#18695=DIRECTION('ref_axis',(1.,0.,0.));
#18696=DIRECTION('',(0.,0.,-1.));
#18697=DIRECTION('',(1.,0.,0.));
#18698=DIRECTION('center_axis',(-1.,0.,0.));
#18699=DIRECTION('ref_axis',(0.,1.,0.));
#18700=DIRECTION('',(0.,0.,-1.));
#18701=DIRECTION('',(0.,1.,0.));
#18702=DIRECTION('center_axis',(0.,-1.,0.));
#18703=DIRECTION('ref_axis',(-1.,0.,0.));
#18704=DIRECTION('',(0.,0.,-1.));
#18705=DIRECTION('',(-1.,0.,0.));
#18706=DIRECTION('center_axis',(1.,0.,0.));
#18707=DIRECTION('ref_axis',(0.,-1.,0.));
#18708=DIRECTION('',(0.,-1.,0.));
#18709=DIRECTION('center_axis',(0.,0.,-1.));
#18710=DIRECTION('ref_axis',(-1.,0.,0.));
#18711=DIRECTION('center_axis',(-1.,0.,0.));
#18712=DIRECTION('ref_axis',(0.,0.,-1.));
#18713=DIRECTION('',(-1.,0.,0.));
#18714=DIRECTION('center_axis',(-1.,0.,0.));
#18715=DIRECTION('ref_axis',(0.,0.,-1.));
#18716=DIRECTION('center_axis',(1.,0.,0.));
#18717=DIRECTION('ref_axis',(0.,0.,-1.));
#18718=DIRECTION('center_axis',(1.,0.,0.));
#18719=DIRECTION('ref_axis',(0.,1.,0.));
#18720=DIRECTION('center_axis',(1.,0.,0.));
#18721=DIRECTION('ref_axis',(0.,1.,0.));
#18722=DIRECTION('',(0.724999433594412,-0.688749461914695,-8.43474823948293E-17));
#18723=DIRECTION('center_axis',(1.,0.,0.));
#18724=DIRECTION('ref_axis',(0.,1.,0.));
#18725=DIRECTION('',(1.,0.,0.));
#18726=DIRECTION('center_axis',(0.,1.,0.));
#18727=DIRECTION('ref_axis',(0.,0.,1.));
#18728=DIRECTION('center_axis',(1.,0.,0.));
#18729=DIRECTION('ref_axis',(0.,0.,-1.));
#18730=DIRECTION('center_axis',(0.,1.,0.));
#18731=DIRECTION('ref_axis',(0.,0.,1.));
#22165=CARTESIAN_POINT('',(0.,0.,0.));
#22166=CARTESIAN_POINT('Origin',(67.75,0.,0.));
#22167=CARTESIAN_POINT('',(67.5,15.2,-1.86146313470398E-15));
#22168=CARTESIAN_POINT('',(67.5,-15.2,-1.86146313470398E-15));
#22169=CARTESIAN_POINT('Origin',(67.5,0.,0.));
#22170=CARTESIAN_POINT('Origin',(67.5,0.,0.));
#22171=CARTESIAN_POINT('',(68.,15.7,1.92269547466134E-15));
#22172=CARTESIAN_POINT('',(67.75,15.45,-1.89207930468266E-15));
#22173=CARTESIAN_POINT('Origin',(68.,0.,0.));
#22174=CARTESIAN_POINT('Origin',(63.95,0.,0.));
#22175=CARTESIAN_POINT('',(60.5,-15.2,-1.86146313470398E-15));
#22176=CARTESIAN_POINT('Origin',(60.5,0.,0.));
#22177=CARTESIAN_POINT('',(63.95,-15.2,-1.86146313470398E-15));
#22178=CARTESIAN_POINT('Origin',(68.,21.05,0.));
#22179=CARTESIAN_POINT('',(68.,-21.05,-2.57788151220518E-15));
#22180=CARTESIAN_POINT('Origin',(68.,0.,0.));
#22181=CARTESIAN_POINT('Origin',(60.25,0.,0.));
#22182=CARTESIAN_POINT('',(60.,-15.7,1.92269547466134E-15));
#22183=CARTESIAN_POINT('Origin',(60.,0.,0.));
#22184=CARTESIAN_POINT('',(60.25,-15.45,1.89207930468266E-15));
#22185=CARTESIAN_POINT('Origin',(60.,-22.,21.));
#22186=CARTESIAN_POINT('',(60.,-20.5,15.1657508881031));
#22187=CARTESIAN_POINT('',(60.,-20.5,-15.1657508881031));
#22188=CARTESIAN_POINT('Origin',(60.,0.,0.));
#22189=CARTESIAN_POINT('',(60.,-20.5,18.));
#22190=CARTESIAN_POINT('',(60.,-20.5,14.75));
#22191=CARTESIAN_POINT('',(60.,20.5,18.));
#22192=CARTESIAN_POINT('',(60.,-22.,18.));
#22193=CARTESIAN_POINT('',(60.,20.5,15.1657508881031));
#22194=CARTESIAN_POINT('',(60.,20.5,14.75));
#22195=CARTESIAN_POINT('',(60.,20.5,-15.1657508881031));
#22196=CARTESIAN_POINT('Origin',(60.,0.,0.));
#22197=CARTESIAN_POINT('',(60.,20.5,-23.5));
#22198=CARTESIAN_POINT('',(60.,20.5,14.75));
#22199=CARTESIAN_POINT('',(60.,9.89949493661168,-23.5));
#22200=CARTESIAN_POINT('',(60.,-22.,-23.5));
#22201=CARTESIAN_POINT('',(60.,-9.89949493661168,-23.5));
#22202=CARTESIAN_POINT('Origin',(60.,0.,0.));
#22203=CARTESIAN_POINT('',(60.,-20.5,-23.5));
#22204=CARTESIAN_POINT('',(60.,-22.,-23.5));
#22205=CARTESIAN_POINT('',(60.,-20.5,14.75));
#22206=CARTESIAN_POINT('Ctrl Pts',(82.590926702435,-21.9972415752925,20.7125564066551));
#22207=CARTESIAN_POINT('Ctrl Pts',(82.5858557493431,-21.9975495316373,20.7099530188172));
#22208=CARTESIAN_POINT('Ctrl Pts',(82.5486931024459,-21.9996721521972,20.6909216201026));
#22209=CARTESIAN_POINT('Ctrl Pts',(82.50785454155,-21.9999804809794,20.67010294536));
#22210=CARTESIAN_POINT('Ctrl Pts',(82.501271349331,-22.,20.6667379107389));
#22211=CARTESIAN_POINT('Ctrl Pts',(82.5,-22.,20.6660888779603));
#22212=CARTESIAN_POINT('Ctrl Pts',(82.4384034141267,-21.9972415752925,21.0089380321363));
#22213=CARTESIAN_POINT('Ctrl Pts',(82.4333341469195,-21.9975495316373,21.0063313683053));
#22214=CARTESIAN_POINT('Ctrl Pts',(82.3962094533413,-21.9996721521972,20.9872262191064));
#22215=CARTESIAN_POINT('Ctrl Pts',(82.3554097305465,-21.9999804809794,20.9663320745804));
#22216=CARTESIAN_POINT('Ctrl Pts',(82.3488347923165,-22.,20.9629510008961));
#22217=CARTESIAN_POINT('Ctrl Pts',(82.3475648606009,-22.,20.9622992134222));
#22218=CARTESIAN_POINT('Ctrl Pts',(82.2858801258184,-21.9972415752925,21.3053196576175));
#22219=CARTESIAN_POINT('Ctrl Pts',(82.2808125444959,-21.9975495316373,21.3027097177933));
#22220=CARTESIAN_POINT('Ctrl Pts',(82.2435888727419,-21.9998742837272,21.2834663188746));
#22221=CARTESIAN_POINT('Ctrl Pts',(82.2029573746821,-21.9998618848641,21.2625298670686));
#22222=CARTESIAN_POINT('Ctrl Pts',(82.1963982353019,-22.,21.2591640910533));
#22223=CARTESIAN_POINT('Ctrl Pts',(82.1951297212018,-22.,21.2585095488841));
#22224=CARTESIAN_POINT('Ctrl Pts',(82.1333568375101,-21.9972415752925,21.6017012830987));
#22225=CARTESIAN_POINT('Ctrl Pts',(82.1282909420722,-21.9975495316373,21.5990880672814));
#22226=CARTESIAN_POINT('Ctrl Pts',(82.091204106178,-21.9996721521972,21.5799093534353));
#22227=CARTESIAN_POINT('Ctrl Pts',(82.0505263223446,-21.9999804809794,21.5587782584214));
#22228=CARTESIAN_POINT('Ctrl Pts',(82.0439616782873,-22.,21.5553771812105));
#22229=CARTESIAN_POINT('Ctrl Pts',(82.0426945818027,-22.,21.5547198843461));
#22230=CARTESIAN_POINT('',(82.5,-22.,20.6660888779603));
#22231=CARTESIAN_POINT('',(82.590926702435,-21.9972415752925,20.7125564066551));
#22232=CARTESIAN_POINT('Ctrl Pts',(82.5,-22.,20.6660888779603));
#22233=CARTESIAN_POINT('Ctrl Pts',(82.5004067990554,-22.,20.6662965517403));
#22234=CARTESIAN_POINT('Ctrl Pts',(82.5008176675242,-21.9999998627569,20.6665063022388));
#22235=CARTESIAN_POINT('Ctrl Pts',(82.5013244717933,-21.999999415258,20.6667650014162));
#22236=CARTESIAN_POINT('Ctrl Pts',(82.5018565166204,-21.9999989454723,20.6670365846832));
#22237=CARTESIAN_POINT('Ctrl Pts',(82.5024940302811,-21.999998138627,20.66736198041));
#22238=CARTESIAN_POINT('Ctrl Pts',(82.5032915692446,-21.9999963885196,20.6677690202808));
#22239=CARTESIAN_POINT('Ctrl Pts',(82.5041416635429,-21.9999945230856,20.6682028828117));
#22240=CARTESIAN_POINT('Ctrl Pts',(82.5051732101651,-21.9999915806081,20.6687293210895));
#22241=CARTESIAN_POINT('Ctrl Pts',(82.5063995751958,-21.999986348417,20.6693551496543));
#22242=CARTESIAN_POINT('Ctrl Pts',(82.507755571728,-21.9999805631631,20.670047130706));
#22243=CARTESIAN_POINT('Ctrl Pts',(82.5093492283813,-21.9999719358723,20.6708603579249));
#22244=CARTESIAN_POINT('Ctrl Pts',(82.5111426325031,-21.9999586133427,20.6717754884718));
#22245=CARTESIAN_POINT('Ctrl Pts',(82.513410125303,-21.9999417689853,20.6729325349515));
#22246=CARTESIAN_POINT('Ctrl Pts',(82.5159957629321,-21.9999172338468,20.6742518848847));
#22247=CARTESIAN_POINT('Ctrl Pts',(82.5187474241439,-21.9998828401205,20.6756559568456));
#22248=CARTESIAN_POINT('Ctrl Pts',(82.5215924246102,-21.9998472797227,20.6771076564103));
#22249=CARTESIAN_POINT('Ctrl Pts',(82.5246090085712,-21.9998011397234,20.6786469157951));
#22250=CARTESIAN_POINT('Ctrl Pts',(82.5276188168876,-21.9997457120971,20.6801828101603));
#22251=CARTESIAN_POINT('Ctrl Pts',(82.5299271169217,-21.9997032032135,20.6813607273707));
#22252=CARTESIAN_POINT('Ctrl Pts',(82.5322304291706,-21.9996553791226,20.682536154127));
#22253=CARTESIAN_POINT('Ctrl Pts',(82.5344785448382,-21.9996036909617,20.683683526565));
#22254=CARTESIAN_POINT('Ctrl Pts',(82.5365092227467,-21.99955700208,20.6847199251347));
#22255=CARTESIAN_POINT('Ctrl Pts',(82.5384943595416,-21.999507235319,20.6857331752724));
#22256=CARTESIAN_POINT('Ctrl Pts',(82.5404338840481,-21.9994549346415,20.6867233017257));
#22257=CARTESIAN_POINT('Ctrl Pts',(82.5422858572142,-21.999404994849,20.6876687332562));
#22258=CARTESIAN_POINT('Ctrl Pts',(82.5440957471635,-21.9993528090371,20.688592827636));
#22259=CARTESIAN_POINT('Ctrl Pts',(82.5459062201873,-21.9992973750888,20.6895174394503));
#22260=CARTESIAN_POINT('Ctrl Pts',(82.5477357383858,-21.9992413580059,20.6904517776694));
#22261=CARTESIAN_POINT('Ctrl Pts',(82.5495738565317,-21.9991817713915,20.6913907373888));
#22262=CARTESIAN_POINT('Ctrl Pts',(82.5514571369584,-21.9991171278643,20.6923530411313));
#22263=CARTESIAN_POINT('Ctrl Pts',(82.5534832655573,-21.9990475810791,20.6933883363034));
#22264=CARTESIAN_POINT('Ctrl Pts',(82.5555612172577,-21.9989721343396,20.6944504217446));
#22265=CARTESIAN_POINT('Ctrl Pts',(82.5576829436322,-21.9988904823282,20.6955351931789));
#22266=CARTESIAN_POINT('Ctrl Pts',(82.5601126519442,-21.9987969780133,20.6967774260145));
#22267=CARTESIAN_POINT('Ctrl Pts',(82.5625990820839,-21.9986952571646,20.6980490614586));
#22268=CARTESIAN_POINT('Ctrl Pts',(82.5650703996693,-21.9985879497336,20.6993133319474));
#22269=CARTESIAN_POINT('Ctrl Pts',(82.5684481340624,-21.99844128465,20.7010413048868));
#22270=CARTESIAN_POINT('Ctrl Pts',(82.5717937906446,-21.9982840158667,20.7027535614366));
#22271=CARTESIAN_POINT('Ctrl Pts',(82.5748462193364,-21.998131517408,20.7043162728701));
#22272=CARTESIAN_POINT('Ctrl Pts',(82.5771355408552,-21.9980171435639,20.7054883064452));
#22273=CARTESIAN_POINT('Ctrl Pts',(82.5792567661969,-21.9979058195173,20.7065745992276));
#22274=CARTESIAN_POINT('Ctrl Pts',(82.5811192797532,-21.9978049480664,20.7075286386024));
#22275=CARTESIAN_POINT('Ctrl Pts',(82.582693322036,-21.9977196998661,20.7083349137086));
#22276=CARTESIAN_POINT('Ctrl Pts',(82.5840820935019,-21.9976420140725,20.7090464755551));
#22277=CARTESIAN_POINT('Ctrl Pts',(82.5852637181514,-21.9975747388251,20.7096520455423));
#22278=CARTESIAN_POINT('Ctrl Pts',(82.5863746838264,-21.9975114865134,20.7102214035612));
#22279=CARTESIAN_POINT('Ctrl Pts',(82.5873020179414,-21.9974574931031,20.7106968005571));
#22280=CARTESIAN_POINT('Ctrl Pts',(82.5880661954622,-21.9974125501066,20.7110886716049));
#22281=CARTESIAN_POINT('Ctrl Pts',(82.5887787608894,-21.9973706425333,20.711454075916));
#22282=CARTESIAN_POINT('Ctrl Pts',(82.5893492752058,-21.9973366162764,20.7117467587141));
#22283=CARTESIAN_POINT('Ctrl Pts',(82.5898336070652,-21.9973075579325,20.7119953098446));
#22284=CARTESIAN_POINT('Ctrl Pts',(82.5902384964647,-21.997283265879,20.7122030924137));
#22285=CARTESIAN_POINT('Ctrl Pts',(82.5905836515537,-21.9972624085941,20.7123802870035));
#22286=CARTESIAN_POINT('Ctrl Pts',(82.590926702435,-21.9972415752925,20.7125564066551));
#22287=CARTESIAN_POINT('',(82.1333568375101,-21.9972415752925,21.6017012830987));
#22288=CARTESIAN_POINT('Ctrl Pts',(82.1333568375101,-21.9972415752925,21.6017012830987));
#22289=CARTESIAN_POINT('Ctrl Pts',(82.2858801258184,-21.9972415752925,21.3053196576175));
#22290=CARTESIAN_POINT('Ctrl Pts',(82.4384034141267,-21.9972415752925,21.0089380321363));
#22291=CARTESIAN_POINT('Ctrl Pts',(82.590926702435,-21.9972415752925,20.7125564066551));
#22292=CARTESIAN_POINT('',(82.0426945818027,-22.,21.5547198843461));
#22293=CARTESIAN_POINT('Ctrl Pts',(82.1333568375101,-21.9972415752925,21.6017012830988));
#22294=CARTESIAN_POINT('Ctrl Pts',(82.1329515455134,-21.9972662130379,21.6014922153299));
#22295=CARTESIAN_POINT('Ctrl Pts',(82.132542196012,-21.9972909606082,21.6012810461369));
#22296=CARTESIAN_POINT('Ctrl Pts',(82.1320373185083,-21.9973212113064,21.6010204716646));
#22297=CARTESIAN_POINT('Ctrl Pts',(82.1315072911072,-21.9973529689088,21.600746916972));
#22298=CARTESIAN_POINT('Ctrl Pts',(82.1308722414686,-21.9973907806112,21.6004190467318));
#22299=CARTESIAN_POINT('Ctrl Pts',(82.1300778406803,-21.9974373473525,21.6000087380818));
#22300=CARTESIAN_POINT('Ctrl Pts',(82.1292310768093,-21.9974869835496,21.5995713838573));
#22301=CARTESIAN_POINT('Ctrl Pts',(82.1282036189947,-21.9975465399409,21.5990405492434));
#22302=CARTESIAN_POINT('Ctrl Pts',(82.1269821372123,-21.9976156171537,21.5984092814532));
#22303=CARTESIAN_POINT('Ctrl Pts',(82.1256314653394,-21.9976920003218,21.5977112475893));
#22304=CARTESIAN_POINT('Ctrl Pts',(82.1240440752437,-21.9977799506085,21.5968906785504));
#22305=CARTESIAN_POINT('Ctrl Pts',(82.1222576842232,-21.9978753225515,21.595966985438));
#22306=CARTESIAN_POINT('Ctrl Pts',(82.1199983913686,-21.9979959418039,21.5947987679398));
#22307=CARTESIAN_POINT('Ctrl Pts',(82.1174219500873,-21.998128176573,21.5934661935896));
#22308=CARTESIAN_POINT('Ctrl Pts',(82.1146799296805,-21.9982606384566,21.5920475040685));
#22309=CARTESIAN_POINT('Ctrl Pts',(82.1118475151583,-21.9983974671111,21.5905820456815));
#22310=CARTESIAN_POINT('Ctrl Pts',(82.1088442875541,-21.998534141336,21.5890277313331));
#22311=CARTESIAN_POINT('Ctrl Pts',(82.1058475042565,-21.9986611634475,21.5874761936605));
#22312=CARTESIAN_POINT('Ctrl Pts',(82.1035482402478,-21.9987586204005,21.5862857856882));
#22313=CARTESIAN_POINT('Ctrl Pts',(82.1012537725383,-21.9988504816478,21.5850975349178));
#22314=CARTESIAN_POINT('Ctrl Pts',(82.0990140514947,-21.9989351541171,21.5839372918622));
#22315=CARTESIAN_POINT('Ctrl Pts',(82.0969908768119,-21.999011640069,21.5828892263531));
#22316=CARTESIAN_POINT('Ctrl Pts',(82.0950128805348,-21.9990823041441,21.5818642778784));
#22317=CARTESIAN_POINT('Ctrl Pts',(82.0930800673691,-21.9991476850095,21.5808624629178));
#22318=CARTESIAN_POINT('Ctrl Pts',(82.0912338430709,-21.9992101368514,21.579905528665));
#22319=CARTESIAN_POINT('Ctrl Pts',(82.0894293434669,-21.999267802336,21.5789699607435));
#22320=CARTESIAN_POINT('Ctrl Pts',(82.0876238971944,-21.9993222687543,21.578033687473));
#22321=CARTESIAN_POINT('Ctrl Pts',(82.0858002202754,-21.9993772851519,21.5770879601041));
#22322=CARTESIAN_POINT('Ctrl Pts',(82.0839675997984,-21.999429270298,21.5761373812524));
#22323=CARTESIAN_POINT('Ctrl Pts',(82.0820895966761,-21.9994789506814,21.5751631199948));
#22324=CARTESIAN_POINT('Ctrl Pts',(82.0800690672747,-21.9995324014313,21.5741149196525));
#22325=CARTESIAN_POINT('Ctrl Pts',(82.0779964515735,-21.9995831102254,21.5730395364255));
#22326=CARTESIAN_POINT('Ctrl Pts',(82.0758798035365,-21.9996302780206,21.5719412139833));
#22327=CARTESIAN_POINT('Ctrl Pts',(82.0734556422703,-21.9996842985002,21.5706833238307));
#22328=CARTESIAN_POINT('Ctrl Pts',(82.0709744016171,-21.999733553745,21.5693956953634));
#22329=CARTESIAN_POINT('Ctrl Pts',(82.0685078519499,-21.9997763068706,21.5681156411538));
#22330=CARTESIAN_POINT('Ctrl Pts',(82.0651377481162,-21.9998347214545,21.5663666734941));
#22331=CARTESIAN_POINT('Ctrl Pts',(82.0617988953356,-21.999880596871,21.564633832814));
#22332=CARTESIAN_POINT('Ctrl Pts',(82.0587521179753,-21.9999134453804,21.5630525919056));
#22333=CARTESIAN_POINT('Ctrl Pts',(82.056467034955,-21.9999380817625,21.5618666612243));
#22334=CARTESIAN_POINT('Ctrl Pts',(82.0543494020555,-21.9999555654168,21.5607676431849));
#22335=CARTESIAN_POINT('Ctrl Pts',(82.0524898204502,-21.9999677944424,21.5598025786458));
#22336=CARTESIAN_POINT('Ctrl Pts',(82.0509182388138,-21.9999781295156,21.5589869770592));
#22337=CARTESIAN_POINT('Ctrl Pts',(82.0495314630858,-21.999984778476,21.5582673069337));
#22338=CARTESIAN_POINT('Ctrl Pts',(82.0483514248692,-21.9999892597033,21.5576549502537));
#22339=CARTESIAN_POINT('Ctrl Pts',(82.0472419209927,-21.9999934730746,21.5570791959257));
#22340=CARTESIAN_POINT('Ctrl Pts',(82.0463156975305,-21.9999957948245,21.5565985785096));
#22341=CARTESIAN_POINT('Ctrl Pts',(82.045552362205,-21.9999972591221,21.5562025087274));
#22342=CARTESIAN_POINT('Ctrl Pts',(82.0448405655344,-21.9999986245536,21.5558331806708));
#22343=CARTESIAN_POINT('Ctrl Pts',(82.0442705930571,-21.9999992450545,21.5555374666851));
#22344=CARTESIAN_POINT('Ctrl Pts',(82.0437866674028,-21.999999599766,21.5552864132347));
#22345=CARTESIAN_POINT('Ctrl Pts',(82.0433821974482,-21.9999998962375,21.5550765802226));
#22346=CARTESIAN_POINT('Ctrl Pts',(82.0430373427831,-22.,21.5548976890519));
#22347=CARTESIAN_POINT('Ctrl Pts',(82.0426945818027,-22.,21.5547198843461));
#22348=CARTESIAN_POINT('',(82.2713472909014,-22.,21.1104043811532));
#22349=CARTESIAN_POINT('Ctrl Pts',(82.1333568375101,-21.9972415752925,21.6017012830987));
#22350=CARTESIAN_POINT('Ctrl Pts',(82.4926054015329,-21.9754028152909,21.7870177866389));
#22351=CARTESIAN_POINT('Ctrl Pts',(83.2880029902013,-21.6082743755756,22.1691719458688));
#22352=CARTESIAN_POINT('Ctrl Pts',(83.5931332643966,-20.8935561866066,22.2906190968596));
#22353=CARTESIAN_POINT('Ctrl Pts',(83.5931332643966,-20.5,22.2906190968596));
#22354=CARTESIAN_POINT('Ctrl Pts',(82.2858801258184,-21.9972415752925,21.3053196576175));
#22355=CARTESIAN_POINT('Ctrl Pts',(82.6452482445491,-21.9754028152909,21.4904038437257));
#22356=CARTESIAN_POINT('Ctrl Pts',(83.4332756664122,-21.6082743755756,21.8868796324069));
#22357=CARTESIAN_POINT('Ctrl Pts',(83.7287555095978,-20.8935561866066,22.0270793979064));
#22358=CARTESIAN_POINT('Ctrl Pts',(83.7287555095978,-20.5,22.0270793979064));
#22359=CARTESIAN_POINT('Ctrl Pts',(82.4384034141267,-21.9972415752925,21.0089380321363));
#22360=CARTESIAN_POINT('Ctrl Pts',(82.7978910875653,-21.9754028152909,21.1937899008126));
#22361=CARTESIAN_POINT('Ctrl Pts',(83.578548342623,-21.6082743755756,21.6045873189449));
#22362=CARTESIAN_POINT('Ctrl Pts',(83.8643777547989,-20.8935561866066,21.7635396989532));
#22363=CARTESIAN_POINT('Ctrl Pts',(83.8643777547989,-20.5,21.7635396989532));
#22364=CARTESIAN_POINT('Ctrl Pts',(82.590926702435,-21.9972415752925,20.7125564066551));
#22365=CARTESIAN_POINT('Ctrl Pts',(82.9505339305815,-21.9754028152909,20.8971759578994));
#22366=CARTESIAN_POINT('Ctrl Pts',(83.7238210188338,-21.6082743755756,21.322295005483));
#22367=CARTESIAN_POINT('Ctrl Pts',(84.,-20.8935561866066,21.5));
#22368=CARTESIAN_POINT('Ctrl Pts',(84.,-20.5,21.5));
#22369=CARTESIAN_POINT('',(84.,-20.5,21.5));
#22370=CARTESIAN_POINT('Ctrl Pts',(82.590926702435,-21.9972415752925,20.7125564066551));
#22371=CARTESIAN_POINT('Ctrl Pts',(82.9505339305815,-21.9754028152909,20.8971759578994));
#22372=CARTESIAN_POINT('Ctrl Pts',(83.7238210188338,-21.6082743755756,21.322295005483));
#22373=CARTESIAN_POINT('Ctrl Pts',(84.,-20.8935561866066,21.5));
#22374=CARTESIAN_POINT('Ctrl Pts',(84.,-20.5,21.5));
#22375=CARTESIAN_POINT('',(83.5931332643966,-20.5,22.2906190968596));
#22376=CARTESIAN_POINT('',(84.,-20.5,21.5));
#22377=CARTESIAN_POINT('Ctrl Pts',(83.5931332643966,-20.5,22.2906190968596));
#22378=CARTESIAN_POINT('Ctrl Pts',(83.5931332643966,-20.8935561866066,22.2906190968596));
#22379=CARTESIAN_POINT('Ctrl Pts',(83.2880029902013,-21.6082743755756,22.1691719458688));
#22380=CARTESIAN_POINT('Ctrl Pts',(82.4926054015329,-21.9754028152909,21.7870177866389));
#22381=CARTESIAN_POINT('Ctrl Pts',(82.1333568375101,-21.9972415752925,21.6017012830987));
#22382=CARTESIAN_POINT('Origin',(83.7965666321983,-22.,21.8953095484298));
#22383=CARTESIAN_POINT('',(84.,-16.3324829710611,21.5));
#22384=CARTESIAN_POINT('',(83.5931332643966,-15.2357572925904,22.2906190968596));
#22385=CARTESIAN_POINT('Origin',(95.0642847487739,0.,0.));
#22386=CARTESIAN_POINT('',(83.5931332643966,-22.,22.2906190968596));
#22387=CARTESIAN_POINT('',(84.,-22.,21.5));
#22388=CARTESIAN_POINT('Origin',(42.,-22.,8.5));
#22389=CARTESIAN_POINT('',(55.5193024198872,-22.,40.5));
#22390=CARTESIAN_POINT('',(58.4153048715835,-22.,38.4314268202169));
#22391=CARTESIAN_POINT('',(6.62132034355964,-22.,40.5));
#22392=CARTESIAN_POINT('',(24.,-22.,40.5));
#22393=CARTESIAN_POINT('',(1.5,-22.,35.3786796564404));
#22394=CARTESIAN_POINT('',(4.68566017177982,-22.,38.5643398282202));
#22395=CARTESIAN_POINT('',(1.5,-22.,-20.3786796564404));
#22396=CARTESIAN_POINT('',(1.5,-22.,-6.25));
#22397=CARTESIAN_POINT('',(4.62132034355965,-22.,-23.5));
#22398=CARTESIAN_POINT('',(6.18566017177982,-22.,-25.0643398282202));
#22399=CARTESIAN_POINT('',(13.5,-22.,-23.5));
#22400=CARTESIAN_POINT('',(56.,-22.,-23.5));
#22401=CARTESIAN_POINT('',(13.5,-22.,18.));
#22402=CARTESIAN_POINT('',(13.5,-22.,-10.75));
#22403=CARTESIAN_POINT('',(18.,-22.,22.5));
#22404=CARTESIAN_POINT('Origin',(18.,-22.,18.));
#22405=CARTESIAN_POINT('',(57.,-22.,22.5));
#22406=CARTESIAN_POINT('',(28.5,-22.,22.5));
#22407=CARTESIAN_POINT('',(61.5,-22.,18.));
#22408=CARTESIAN_POINT('Origin',(57.,-22.,18.));
#22409=CARTESIAN_POINT('',(61.5,-22.,15.6524758424985));
#22410=CARTESIAN_POINT('',(61.5,-22.,14.75));
#22411=CARTESIAN_POINT('',(82.5,-22.,15.6524758424985));
#22412=CARTESIAN_POINT('',(75.5,-22.,15.6524758424985));
#22413=CARTESIAN_POINT('',(82.5,-22.,15.25));
#22414=CARTESIAN_POINT('Origin',(58.4153048715835,-20.5,38.4314268202169));
#22415=CARTESIAN_POINT('',(56.3911597104659,-20.5,41.7206002068101));
#22416=CARTESIAN_POINT('',(59.2871621621622,-20.5,39.652027027027));
#22417=CARTESIAN_POINT('Origin',(55.5193024198872,-20.5,40.5));
#22418=CARTESIAN_POINT('Origin',(56.,-22.,42.));
#22419=CARTESIAN_POINT('',(83.3718572905786,15.0019020194829,22.4486733638724));
#22420=CARTESIAN_POINT('Origin',(114.8,0.,0.));
#22421=CARTESIAN_POINT('',(83.3718572905786,20.5,22.4486733638724));
#22422=CARTESIAN_POINT('',(83.3718572905786,-22.,22.4486733638724));
#22423=CARTESIAN_POINT('',(56.3911597104659,20.5,41.7206002068101));
#22424=CARTESIAN_POINT('',(59.2871621621622,20.5,39.652027027027));
#22425=CARTESIAN_POINT('',(56.3911597104659,-22.,41.7206002068101));
#22426=CARTESIAN_POINT('Ctrl Pts',(4.54678558986685,19.8682455202995,-24.9981470456841));
#22427=CARTESIAN_POINT('Ctrl Pts',(4.55093583868358,19.8641612816606,-24.9983535259319));
#22428=CARTESIAN_POINT('Ctrl Pts',(4.58143737374893,19.8342243880485,-24.9997804759391));
#22429=CARTESIAN_POINT('Ctrl Pts',(4.61489089919229,19.8015972979556,-24.9999871969247));
#22430=CARTESIAN_POINT('Ctrl Pts',(4.62027734084719,19.7963354971355,-25.));
#22431=CARTESIAN_POINT('Ctrl Pts',(4.62132034355965,19.7953186364093,-25.));
#22432=CARTESIAN_POINT('Ctrl Pts',(4.7822153343313,20.1036752647639,-24.9981470456841));
#22433=CARTESIAN_POINT('Ctrl Pts',(4.78634357975541,20.0995690227324,-24.9983535259319));
#22434=CARTESIAN_POINT('Ctrl Pts',(4.81661719703365,20.0694042113332,-24.9997804759391));
#22435=CARTESIAN_POINT('Ctrl Pts',(4.8498425300617,20.036548928825,-24.9999871969247));
#22436=CARTESIAN_POINT('Ctrl Pts',(4.85517984270618,20.0312379989945,-25.));
#22437=CARTESIAN_POINT('Ctrl Pts',(4.85621413142322,20.0302124242728,-25.));
#22438=CARTESIAN_POINT('Ctrl Pts',(5.01764507879574,20.3391050092283,-24.9981470456841));
#22439=CARTESIAN_POINT('Ctrl Pts',(5.02175132082723,20.3349767638042,-24.9983535259319));
#22440=CARTESIAN_POINT('Ctrl Pts',(5.05191613222637,20.304526175821,-25.0000202744737));
#22441=CARTESIAN_POINT('Ctrl Pts',(5.08477141473465,20.271453204594,-24.9998345971494));
#22442=CARTESIAN_POINT('Ctrl Pts',(5.09008234456518,20.2661405008535,-25.));
#22443=CARTESIAN_POINT('Ctrl Pts',(5.0911079192868,20.2651062121364,-25.));
#22444=CARTESIAN_POINT('Ctrl Pts',(5.25307482326019,20.5745347536928,-24.9981470456841));
#22445=CARTESIAN_POINT('Ctrl Pts',(5.25715906189905,20.5703845048761,-24.9983535259319));
#22446=CARTESIAN_POINT('Ctrl Pts',(5.28709595551109,20.5398829698107,-24.9997804759391));
#22447=CARTESIAN_POINT('Ctrl Pts',(5.31972304560406,20.5064294443674,-24.9999871969247));
#22448=CARTESIAN_POINT('Ctrl Pts',(5.32498484642417,20.5010430027125,-25.));
#22449=CARTESIAN_POINT('Ctrl Pts',(5.32600170715038,20.5,-25.));
#22450=CARTESIAN_POINT('',(4.62132034355965,19.7953186364093,-25.));
#22451=CARTESIAN_POINT('',(4.54678558986685,19.8682455202995,-24.9981470456841));
#22452=CARTESIAN_POINT('Ctrl Pts',(4.62132034355965,19.7953186364093,-25.));
#22453=CARTESIAN_POINT('Ctrl Pts',(4.62098833704959,19.7956423214552,-25.));
#22454=CARTESIAN_POINT('Ctrl Pts',(4.62065306038901,19.7959691994142,-24.9999999083843));
#22455=CARTESIAN_POINT('Ctrl Pts',(4.62024024126657,19.7963717921936,-24.9999996111263));
#22456=CARTESIAN_POINT('Ctrl Pts',(4.61980697903812,19.7967943216629,-24.9999992991479));
#22457=CARTESIAN_POINT('Ctrl Pts',(4.61928851221717,19.7973000472878,-24.9999987638439));
#22458=CARTESIAN_POINT('Ctrl Pts',(4.61864053809611,19.7979322315752,-24.9999976062123));
#22459=CARTESIAN_POINT('Ctrl Pts',(4.61795018430504,19.7986057628248,-24.9999963728678));
#22460=CARTESIAN_POINT('Ctrl Pts',(4.61711311377486,19.7994225566992,-24.9999944297595));
#22461=CARTESIAN_POINT('Ctrl Pts',(4.61611808610815,19.8003936022613,-24.999990978812));
#22462=CARTESIAN_POINT('Ctrl Pts',(4.61501963958223,19.8014655740868,-24.999987169188));
#22463=CARTESIAN_POINT('Ctrl Pts',(4.61372910964003,19.8027251227113,-24.9999814945831));
#22464=CARTESIAN_POINT('Ctrl Pts',(4.61227623408374,19.8041432486014,-24.9999727344468));
#22465=CARTESIAN_POINT('Ctrl Pts',(4.61045329055158,19.8059225912354,-24.9999617429798));
#22466=CARTESIAN_POINT('Ctrl Pts',(4.60837566715098,19.8079507006083,-24.9999457782408));
#22467=CARTESIAN_POINT('Ctrl Pts',(4.60616166416588,19.8101121911254,-24.9999234028573));
#22468=CARTESIAN_POINT('Ctrl Pts',(4.60381355266282,19.8124046093294,-24.9998996721325));
#22469=CARTESIAN_POINT('Ctrl Pts',(4.60131688796196,19.8148423226041,-24.9998686879986));
#22470=CARTESIAN_POINT('Ctrl Pts',(4.59882328102637,19.817277508365,-24.9998312845708));
#22471=CARTESIAN_POINT('Ctrl Pts',(4.59693379067582,19.8191227310148,-24.999802942728));
#22472=CARTESIAN_POINT('Ctrl Pts',(4.59504687759637,19.8209657010644,-24.9997710160886));
#22473=CARTESIAN_POINT('Ctrl Pts',(4.59320445521053,19.8227656108414,-24.9997364757924));
#22474=CARTESIAN_POINT('Ctrl Pts',(4.59154190291722,19.8243898009026,-24.9997053075603));
#22475=CARTESIAN_POINT('Ctrl Pts',(4.5899159891667,19.8259785263526,-24.9996720606843));
#22476=CARTESIAN_POINT('Ctrl Pts',(4.58832795537129,19.8275306848797,-24.9996371235474));
#22477=CARTESIAN_POINT('Ctrl Pts',(4.58676097332109,19.8290622672415,-24.9996026495542));
#22478=CARTESIAN_POINT('Ctrl Pts',(4.58523154624858,19.8305575877079,-24.9995665836662));
#22479=CARTESIAN_POINT('Ctrl Pts',(4.58370227592527,19.8320533055383,-24.9995282194702));
#22480=CARTESIAN_POINT('Ctrl Pts',(4.58221111704353,19.8335117480997,-24.9994908113608));
#22481=CARTESIAN_POINT('Ctrl Pts',(4.58071342303859,19.8349771101062,-24.999451043943));
#22482=CARTESIAN_POINT('Ctrl Pts',(4.57917937054696,19.8364785839886,-24.9994079292819));
#22483=CARTESIAN_POINT('Ctrl Pts',(4.57753054138005,19.8380923970388,-24.9993615888138));
#22484=CARTESIAN_POINT('Ctrl Pts',(4.5758400682372,19.8397475771906,-24.999311351025));
#22485=CARTESIAN_POINT('Ctrl Pts',(4.57411385800763,19.8414382892535,-24.9992569985569));
#22486=CARTESIAN_POINT('Ctrl Pts',(4.57214165480933,19.8433699356316,-24.9991949006098));
#22487=CARTESIAN_POINT('Ctrl Pts',(4.57012334014877,19.8453474383937,-24.9991273806813));
#22488=CARTESIAN_POINT('Ctrl Pts',(4.56811545869005,19.8473152862887,-24.9990561164366));
#22489=CARTESIAN_POINT('Ctrl Pts',(4.56533443804158,19.8500408583613,-24.9989574117372));
#22490=CARTESIAN_POINT('Ctrl Pts',(4.562576391132,19.852745017667,-24.9988513941288));
#22491=CARTESIAN_POINT('Ctrl Pts',(4.5600578537522,19.855215144939,-24.9987484469859));
#22492=CARTESIAN_POINT('Ctrl Pts',(4.55816895071736,19.8570677403929,-24.9986712366287));
#22493=CARTESIAN_POINT('Ctrl Pts',(4.55641746154057,19.8587860498669,-24.9985960052401));
#22494=CARTESIAN_POINT('Ctrl Pts',(4.55487916244497,19.8602955926206,-24.9985278006938));
#22495=CARTESIAN_POINT('Ctrl Pts',(4.55359016866188,19.8615604904745,-24.9984706497558));
#22496=CARTESIAN_POINT('Ctrl Pts',(4.55245123366914,19.8626784402,-24.9984184962121));
#22497=CARTESIAN_POINT('Ctrl Pts',(4.55148064564489,19.8636314053933,-24.9983732567672));
#22498=CARTESIAN_POINT('Ctrl Pts',(4.55056811294028,19.8645273693692,-24.9983307233009));
#22499=CARTESIAN_POINT('Ctrl Pts',(4.54980480757313,19.865277085181,-24.9982943388109));
#22500=CARTESIAN_POINT('Ctrl Pts',(4.54917498181042,19.8658959318917,-24.9982640110401));
#22501=CARTESIAN_POINT('Ctrl Pts',(4.54858795079092,19.8664727298523,-24.9982357439491));
#22502=CARTESIAN_POINT('Ctrl Pts',(4.54811702674687,19.8669356913585,-24.9982127465679));
#22503=CARTESIAN_POINT('Ctrl Pts',(4.54771804473987,19.8673281021022,-24.9981931456286));
#22504=CARTESIAN_POINT('Ctrl Pts',(4.54737031074586,19.8676701088915,-24.9981760623697));
#22505=CARTESIAN_POINT('Ctrl Pts',(4.54707695328725,19.8679587910473,-24.9981615413912));
#22506=CARTESIAN_POINT('Ctrl Pts',(4.54678558986685,19.8682455202995,-24.9981470456841));
#22507=CARTESIAN_POINT('',(5.25307482326019,20.5745347536928,-24.9981470456841));
#22508=CARTESIAN_POINT('Ctrl Pts',(5.25307482326019,20.5745347536928,-24.9981470456841));
#22509=CARTESIAN_POINT('Ctrl Pts',(5.01764507879574,20.3391050092283,-24.9981470456841));
#22510=CARTESIAN_POINT('Ctrl Pts',(4.7822153343313,20.1036752647639,-24.9981470456841));
#22511=CARTESIAN_POINT('Ctrl Pts',(4.54678558986685,19.8682455202995,-24.9981470456841));
#22512=CARTESIAN_POINT('',(5.32600170715038,20.5,-25.));
#22513=CARTESIAN_POINT('Ctrl Pts',(5.25307482326019,20.5745347536928,-24.9981470456841));
#22514=CARTESIAN_POINT('Ctrl Pts',(5.25339985886691,20.5742044648039,-24.9981634779836));
#22515=CARTESIAN_POINT('Ctrl Pts',(5.2537280933634,20.5738709111413,-24.9981799817513));
#22516=CARTESIAN_POINT('Ctrl Pts',(5.25413216335514,20.5734600252166,-24.9982001283858));
#22517=CARTESIAN_POINT('Ctrl Pts',(5.25455624459622,20.5730287904889,-24.9982212727665));
#22518=CARTESIAN_POINT('Ctrl Pts',(5.25506365516221,20.572512581772,-24.9982464226455));
#22519=CARTESIAN_POINT('Ctrl Pts',(5.2556977141089,20.5718671927797,-24.9982773797271));
#22520=CARTESIAN_POINT('Ctrl Pts',(5.25637324645706,20.5711795892946,-24.9983103616922));
#22521=CARTESIAN_POINT('Ctrl Pts',(5.25719225799349,20.5703456377491,-24.9983499179323));
#22522=CARTESIAN_POINT('Ctrl Pts',(5.25816572676123,20.5693540673989,-24.9983958133068));
#22523=CARTESIAN_POINT('Ctrl Pts',(5.25924039301158,20.5682594178061,-24.9984464797602));
#22524=CARTESIAN_POINT('Ctrl Pts',(5.26050289280568,20.5669730879005,-24.9985048239997));
#22525=CARTESIAN_POINT('Ctrl Pts',(5.26192412261039,20.5655246259075,-24.9985681577425));
#22526=CARTESIAN_POINT('Ctrl Pts',(5.26370752556061,20.5637070511684,-24.9986476308744));
#22527=CARTESIAN_POINT('Ctrl Pts',(5.26573998138134,20.5616350783528,-24.9987348006106));
#22528=CARTESIAN_POINT('Ctrl Pts',(5.26790573837352,20.5594265093687,-24.9988223677222));
#22529=CARTESIAN_POINT('Ctrl Pts',(5.27020197977311,20.5570848766032,-24.998915210653));
#22530=CARTESIAN_POINT('Ctrl Pts',(5.27264332828516,20.5545945239351,-24.9990082175786));
#22531=CARTESIAN_POINT('Ctrl Pts',(5.2750816169699,20.5521063655077,-24.9990947023699));
#22532=CARTESIAN_POINT('Ctrl Pts',(5.27692945702648,20.5502207320148,-24.9991602442652));
#22533=CARTESIAN_POINT('Ctrl Pts',(5.27877473625192,20.548337181907,-24.9992220998817));
#22534=CARTESIAN_POINT('Ctrl Pts',(5.28057649496845,20.5464974338248,-24.999279156344));
#22535=CARTESIAN_POINT('Ctrl Pts',(5.28220237330072,20.5448372744947,-24.9993306431857));
#22536=CARTESIAN_POINT('Ctrl Pts',(5.28379241057199,20.5432131948601,-24.9993782510764));
#22537=CARTESIAN_POINT('Ctrl Pts',(5.28534543187148,20.5416263520351,-24.9994223043613));
#22538=CARTESIAN_POINT('Ctrl Pts',(5.28687822685119,20.5400601760164,-24.9994657839028));
#22539=CARTESIAN_POINT('Ctrl Pts',(5.28837430276488,20.5385309483966,-24.9995058211122));
#22540=CARTESIAN_POINT('Ctrl Pts',(5.28987033506272,20.5370012069583,-24.999543567451));
#22541=CARTESIAN_POINT('Ctrl Pts',(5.29132872010489,20.5355099610573,-24.9995803639132));
#22542=CARTESIAN_POINT('Ctrl Pts',(5.29279360477615,20.5340115437723,-24.9996151417452));
#22543=CARTESIAN_POINT('Ctrl Pts',(5.29429419368321,20.5324761755474,-24.9996483914644));
#22544=CARTESIAN_POINT('Ctrl Pts',(5.29590707598065,20.5308259112954,-24.9996841293559));
#22545=CARTESIAN_POINT('Ctrl Pts',(5.29756085615442,20.5291333163862,-24.9997180535011));
#22546=CARTESIAN_POINT('Ctrl Pts',(5.29924977607504,20.5274044083941,-24.999749645241));
#22547=CARTESIAN_POINT('Ctrl Pts',(5.30117946913945,20.5254290265417,-24.9997857407128));
#22548=CARTESIAN_POINT('Ctrl Pts',(5.30315451227523,20.5234067749386,-24.9998187134049));
#22549=CARTESIAN_POINT('Ctrl Pts',(5.30511956577291,20.5213944706428,-24.9998474177815));
#22550=CARTESIAN_POINT('Ctrl Pts',(5.30784086271432,20.5186077386114,-24.9998871689295));
#22551=CARTESIAN_POINT('Ctrl Pts',(5.31054011508801,20.5158430430512,-24.9999184562551));
#22552=CARTESIAN_POINT('Ctrl Pts',(5.3130053286776,20.5133177855987,-24.9999408776971));
#22553=CARTESIAN_POINT('Ctrl Pts',(5.31485423886979,20.5114238425093,-24.9999576937786));
#22554=CARTESIAN_POINT('Ctrl Pts',(5.31656886411985,20.5096672835416,-24.9999696412555));
#22555=CARTESIAN_POINT('Ctrl Pts',(5.31807494917383,20.5081242380259,-24.9999779987575));
#22556=CARTESIAN_POINT('Ctrl Pts',(5.31933697354538,20.5068312426256,-24.9999850019285));
#22557=CARTESIAN_POINT('Ctrl Pts',(5.32045220380261,20.5056885414075,-24.9999895296818));
#22558=CARTESIAN_POINT('Ctrl Pts',(5.32140268042815,20.5047145553013,-24.9999925909711));
#22559=CARTESIAN_POINT('Ctrl Pts',(5.32229631396741,20.5037988182617,-24.9999954691806));
#22560=CARTESIAN_POINT('Ctrl Pts',(5.32304390109983,20.5030326389375,-24.9999970676595));
#22561=CARTESIAN_POINT('Ctrl Pts',(5.32366082469884,20.5024002743131,-24.9999980795598));
#22562=CARTESIAN_POINT('Ctrl Pts',(5.32423583584433,20.501810871172,-24.9999990227139));
#22563=CARTESIAN_POINT('Ctrl Pts',(5.32469718707828,20.5013378687583,-24.9999994569353));
#22564=CARTESIAN_POINT('Ctrl Pts',(5.32508810907333,20.5009369959301,-24.9999997073462));
#22565=CARTESIAN_POINT('Ctrl Pts',(5.32542876905438,20.5005876645244,-24.999999925561));
#22566=CARTESIAN_POINT('Ctrl Pts',(5.3257162121543,20.5002928346505,-25.));
#22567=CARTESIAN_POINT('Ctrl Pts',(5.32600170715039,20.5,-25.));
#22568=CARTESIAN_POINT('',(4.97366102535501,20.1476593182046,-25.));
#22569=CARTESIAN_POINT('Ctrl Pts',(0.00185295431591348,20.5745347536928,
-19.7469251767398));
#22570=CARTESIAN_POINT('Ctrl Pts',(0.00164647406805663,20.5703845048761,
-19.742840938101));
#22571=CARTESIAN_POINT('Ctrl Pts',(0.000218999411820001,20.5398627220639,
-19.7128841548999));
#22572=CARTESIAN_POINT('Ctrl Pts',(1.27370737248938E-5,20.5064246274686,
-19.6802722284864));
#22573=CARTESIAN_POINT('Ctrl Pts',(-9.64971355100933E-20,20.5010430027125,
-19.6750151535758));
#22574=CARTESIAN_POINT('Ctrl Pts',(0.,20.5,-19.6739982928496));
#22575=CARTESIAN_POINT('Ctrl Pts',(0.00185295431591376,20.3391050092284,
-19.9823549212043));
#22576=CARTESIAN_POINT('Ctrl Pts',(0.00164647406805682,20.3349767638042,
-19.9782486791728));
#22577=CARTESIAN_POINT('Ctrl Pts',(0.000218999411820078,20.3046828987792,
-19.9480639781846));
#22578=CARTESIAN_POINT('Ctrl Pts',(1.27370737249021E-5,20.2714729965992,
-19.9152238593558));
#22579=CARTESIAN_POINT('Ctrl Pts',(-6.62449705573466E-20,20.2661405008535,
-19.9099176554348));
#22580=CARTESIAN_POINT('Ctrl Pts',(0.,20.2651062121364,-19.9088920807132));
#22581=CARTESIAN_POINT('Ctrl Pts',(0.00185295431591403,20.1036752647639,
-20.2177846656687));
#22582=CARTESIAN_POINT('Ctrl Pts',(0.00164647406805702,20.0995690227324,
-20.2136564202446));
#22583=CARTESIAN_POINT('Ctrl Pts',(-1.76372974816777E-5,20.0693843217443,
-20.1831854192229));
#22584=CARTESIAN_POINT('Ctrl Pts',(0.000166089722694393,20.0365442029154,
-20.150128023312));
#22585=CARTESIAN_POINT('Ctrl Pts',(-2.83060097038847E-20,20.0312379989945,
-20.1448201572938));
#22586=CARTESIAN_POINT('Ctrl Pts',(0.,20.0302124242728,-20.1437858685768));
#22587=CARTESIAN_POINT('Ctrl Pts',(0.00185295431591431,19.8682455202995,
-20.4532144101331));
#22588=CARTESIAN_POINT('Ctrl Pts',(0.00164647406805721,19.8641612816606,
-20.4490641613164));
#22589=CARTESIAN_POINT('Ctrl Pts',(0.00021899941182044,19.8342044984596,
-20.4185423785043));
#22590=CARTESIAN_POINT('Ctrl Pts',(1.27370737248456E-5,19.801592572046,
-20.385104283909));
#22591=CARTESIAN_POINT('Ctrl Pts',(0.,19.7963354971355,-20.3797226591528));
#22592=CARTESIAN_POINT('Ctrl Pts',(0.,19.7953186364093,-20.3786796564404));
#22593=CARTESIAN_POINT('',(0.,20.5,-19.6739982928496));
#22594=CARTESIAN_POINT('',(0.00185295431591348,20.5745347536928,-19.7469251767398));
#22595=CARTESIAN_POINT('Ctrl Pts',(-1.33226762955019E-15,20.5,-19.6739982928496));
#22596=CARTESIAN_POINT('Ctrl Pts',(-1.33226762955019E-15,20.5003320065101,
-19.6743219778956));
#22597=CARTESIAN_POINT('Ctrl Pts',(9.16157061043807E-8,20.5006672831706,
-19.6746488558546));
#22598=CARTESIAN_POINT('Ctrl Pts',(3.88873703682791E-7,20.5010801022931,
-19.6750514486339));
#22599=CARTESIAN_POINT('Ctrl Pts',(7.00852135530467E-7,20.5015133645215,
-19.6754739781033));
#22600=CARTESIAN_POINT('Ctrl Pts',(1.2361561089926E-6,20.5020318313425,
-19.6759797037281));
#22601=CARTESIAN_POINT('Ctrl Pts',(2.39378768296383E-6,20.5026798054635,
-19.6766118880155));
#22602=CARTESIAN_POINT('Ctrl Pts',(3.62713222530517E-6,20.5033701592546,
-19.6772854192651));
#22603=CARTESIAN_POINT('Ctrl Pts',(5.57024050657816E-6,20.5042072297849,
-19.6781022131396));
#22604=CARTESIAN_POINT('Ctrl Pts',(9.02118799039897E-6,20.5052022574516,
-19.6790732587018));
#22605=CARTESIAN_POINT('Ctrl Pts',(1.28308119852926E-5,20.5063007039776,
-19.6801452305273));
#22606=CARTESIAN_POINT('Ctrl Pts',(1.85054169170547E-5,20.5075912339199,
-19.6814047791519));
#22607=CARTESIAN_POINT('Ctrl Pts',(2.72655532085331E-5,20.5090441094763,
-19.6828229050421));
#22608=CARTESIAN_POINT('Ctrl Pts',(3.82570202503681E-5,20.5108670530085,
-19.6846022476762));
#22609=CARTESIAN_POINT('Ctrl Pts',(5.42217591519492E-5,20.5129446764091,
-19.6866303570491));
#22610=CARTESIAN_POINT('Ctrl Pts',(7.65971426985868E-5,20.5151586793942,
-19.6887918475662));
#22611=CARTESIAN_POINT('Ctrl Pts',(0.000100327867472851,20.5175067908972,
-19.6910842657702));
#22612=CARTESIAN_POINT('Ctrl Pts',(0.000131312001377887,20.520003455598,
-19.6935219790447));
#22613=CARTESIAN_POINT('Ctrl Pts',(0.000168715429175847,20.5224970625335,
-19.6959571648056));
#22614=CARTESIAN_POINT('Ctrl Pts',(0.00019705727202824,20.524386552884,
-19.6978023874553));
#22615=CARTESIAN_POINT('Ctrl Pts',(0.000228983911360227,20.5262734659634,
-19.6996453575049));
#22616=CARTESIAN_POINT('Ctrl Pts',(0.000263524207557708,20.5281158883493,
-19.701445267282));
#22617=CARTESIAN_POINT('Ctrl Pts',(0.000294692439715454,20.5297784406426,
-19.7030694573431));
#22618=CARTESIAN_POINT('Ctrl Pts',(0.000327939315699018,20.5314043543931,
-19.704658182793));
#22619=CARTESIAN_POINT('Ctrl Pts',(0.00036287645256472,20.5329923881885,
-19.7062103413201));
#22620=CARTESIAN_POINT('Ctrl Pts',(0.000397350445821907,20.5345593702387,
-19.707741923682));
#22621=CARTESIAN_POINT('Ctrl Pts',(0.00043341633385059,20.5360887973112,
-19.7092372441484));
#22622=CARTESIAN_POINT('Ctrl Pts',(0.000471780529807564,20.5376180676346,
-19.7107329619788));
#22623=CARTESIAN_POINT('Ctrl Pts',(0.000509188639198179,20.5391092265163,
-19.7121914045402));
#22624=CARTESIAN_POINT('Ctrl Pts',(0.000548956057017146,20.5406069205213,
-19.7136567665468));
#22625=CARTESIAN_POINT('Ctrl Pts',(0.000592070718070437,20.542140973013,
-19.7151582404293));
#22626=CARTESIAN_POINT('Ctrl Pts',(0.000638411186244535,20.5437898021799,
-19.7167720534795));
#22627=CARTESIAN_POINT('Ctrl Pts',(0.000688648974965052,20.5454802753228,
-19.7184272336313));
#22628=CARTESIAN_POINT('Ctrl Pts',(0.000743001443115787,20.5472064855524,
-19.7201179456942));
#22629=CARTESIAN_POINT('Ctrl Pts',(0.000805099390218029,20.5491786887507,
-19.7220495920723));
#22630=CARTESIAN_POINT('Ctrl Pts',(0.000872619318741684,20.5511970034113,
-19.7240270948345));
#22631=CARTESIAN_POINT('Ctrl Pts',(0.000943883563405024,20.5532048848701,
-19.7259949427295));
#22632=CARTESIAN_POINT('Ctrl Pts',(0.0010425882628478,20.5559859055185,
-19.7287205148021));
#22633=CARTESIAN_POINT('Ctrl Pts',(0.00114860587122066,20.558743952428,
-19.7314246741078));
#22634=CARTESIAN_POINT('Ctrl Pts',(0.00125155301412994,20.5612624898078,
-19.7338948013796));
#22635=CARTESIAN_POINT('Ctrl Pts',(0.00132876337131189,20.5631513928426,
-19.7357473968336));
#22636=CARTESIAN_POINT('Ctrl Pts',(0.00140399475990964,20.5649028820193,
-19.7374657063075));
#22637=CARTESIAN_POINT('Ctrl Pts',(0.00147219930624476,20.5664411811149,
-19.7389752490611));
#22638=CARTESIAN_POINT('Ctrl Pts',(0.00152935024422438,20.567730174898,
-19.7402401469151));
#22639=CARTESIAN_POINT('Ctrl Pts',(0.00158150378788142,20.5688691098907,
-19.7413580966406));
#22640=CARTESIAN_POINT('Ctrl Pts',(0.00162674323279743,20.5698396979149,
-19.7423110618338));
#22641=CARTESIAN_POINT('Ctrl Pts',(0.00166927669910059,20.5707522306195,
-19.7432070258097));
#22642=CARTESIAN_POINT('Ctrl Pts',(0.00170566118909408,20.5715155359867,
-19.7439567416215));
#22643=CARTESIAN_POINT('Ctrl Pts',(0.00173598895987004,20.5721453617494,
-19.7445755883322));
#22644=CARTESIAN_POINT('Ctrl Pts',(0.00176425605094743,20.5727323927688,
-19.7451523862928));
#22645=CARTESIAN_POINT('Ctrl Pts',(0.001787253432131,20.5732033168129,-19.7456153477989));
#22646=CARTESIAN_POINT('Ctrl Pts',(0.0018068543714278,20.5736022988199,
-19.7460077585426));
#22647=CARTESIAN_POINT('Ctrl Pts',(0.0018239376302916,20.5739500328138,
-19.7463497653319));
#22648=CARTESIAN_POINT('Ctrl Pts',(0.00183845860880921,20.5742433902724,
-19.7466384474877));
#22649=CARTESIAN_POINT('Ctrl Pts',(0.00185295431591337,20.5745347536928,
-19.7469251767398));
#22650=CARTESIAN_POINT('',(0.00185295431591431,19.8682455202995,-20.4532144101331));
#22651=CARTESIAN_POINT('Ctrl Pts',(0.00185295431591431,19.8682455202995,
-20.4532144101331));
#22652=CARTESIAN_POINT('Ctrl Pts',(0.00185295431591403,20.1036752647639,
-20.2177846656687));
#22653=CARTESIAN_POINT('Ctrl Pts',(0.00185295431591376,20.3391050092284,
-19.9823549212043));
#22654=CARTESIAN_POINT('Ctrl Pts',(0.00185295431591348,20.5745347536928,
-19.7469251767398));
#22655=CARTESIAN_POINT('',(0.,19.7953186364093,-20.3786796564404));
#22656=CARTESIAN_POINT('Ctrl Pts',(0.00185295431591403,19.8682455202995,
-20.4532144101332));
#22657=CARTESIAN_POINT('Ctrl Pts',(0.0018365220163917,19.8679204846928,
-20.4528841212442));
#22658=CARTESIAN_POINT('Ctrl Pts',(0.0018200182487141,19.8675922501963,
-20.4525505675817));
#22659=CARTESIAN_POINT('Ctrl Pts',(0.00179987161422024,19.8671881802045,
-20.452139681657));
#22660=CARTESIAN_POINT('Ctrl Pts',(0.00177872723345861,19.8667640989635,
-20.4517084469293));
#22661=CARTESIAN_POINT('Ctrl Pts',(0.00175357735450232,19.8662566883975,
-20.4511922382125));
#22662=CARTESIAN_POINT('Ctrl Pts',(0.00172262027288483,19.8656226294509,
-20.4505468492202));
#22663=CARTESIAN_POINT('Ctrl Pts',(0.00168963830780533,19.8649470971028,
-20.4498592457351));
#22664=CARTESIAN_POINT('Ctrl Pts',(0.00165008206768198,19.8641280855664,
-20.4490252941897));
#22665=CARTESIAN_POINT('Ctrl Pts',(0.00160418669325102,19.8631546167987,
-20.4480337238395));
#22666=CARTESIAN_POINT('Ctrl Pts',(0.00155352023986771,19.8620799505485,
-20.4469390742469));
#22667=CARTESIAN_POINT('Ctrl Pts',(0.00149517600032736,19.8608174507546,
-20.4456527443415));
#22668=CARTESIAN_POINT('Ctrl Pts',(0.00143184225756587,19.8593962209502,
-20.4442042823488));
#22669=CARTESIAN_POINT('Ctrl Pts',(0.00135236912569878,19.8576128180005,
-20.4423867076102));
#22670=CARTESIAN_POINT('Ctrl Pts',(0.0012651993894486,19.8555803621803,
-20.4403147347952));
#22671=CARTESIAN_POINT('Ctrl Pts',(0.00117763227794754,19.8534146051887,
-20.4381061658117));
#22672=CARTESIAN_POINT('Ctrl Pts',(0.00108478934705518,19.8511183637887,
-20.4357645330458));
#22673=CARTESIAN_POINT('Ctrl Pts',(0.000991782421426017,19.8486770152762,
-20.4332741803772));
#22674=CARTESIAN_POINT('Ctrl Pts',(0.000905297630115376,19.8462387265909,
-20.4307860219493));
#22675=CARTESIAN_POINT('Ctrl Pts',(0.00083975573483102,19.8443908865342,
-20.4289003884562));
#22676=CARTESIAN_POINT('Ctrl Pts',(0.000777900118314327,19.8425456073086,
-20.4270168383482));
#22677=CARTESIAN_POINT('Ctrl Pts',(0.000720843655976244,19.8407438485919,
-20.4251770902658));
#22678=CARTESIAN_POINT('Ctrl Pts',(0.000669356814273844,19.8391179702596,
-20.4235169309357));
#22679=CARTESIAN_POINT('Ctrl Pts',(0.000621748923652178,19.8375279329883,
-20.4218928513011));
#22680=CARTESIAN_POINT('Ctrl Pts',(0.000577695638684927,19.8359749116888,
-20.4203060084761));
#22681=CARTESIAN_POINT('Ctrl Pts',(0.000534216097193185,19.8344421167093,
-20.4187398324576));
#22682=CARTESIAN_POINT('Ctrl Pts',(0.000494178887846744,19.8329460407958,
-20.417210604838));
#22683=CARTESIAN_POINT('Ctrl Pts',(0.000456432549044816,19.8314500084981,
-20.4156808633999));
#22684=CARTESIAN_POINT('Ctrl Pts',(0.000419636086835154,19.829991623456,
-20.4141896174989));
#22685=CARTESIAN_POINT('Ctrl Pts',(0.000384858254870382,19.8285267387848,
-20.412691200214));
#22686=CARTESIAN_POINT('Ctrl Pts',(0.000351608535610337,19.8270261498778,
-20.411155831989));
#22687=CARTESIAN_POINT('Ctrl Pts',(0.000315870644081551,19.8254132675804,
-20.4095055677372));
#22688=CARTESIAN_POINT('Ctrl Pts',(0.000281946498895475,19.8237594874066,
-20.407812972828));
#22689=CARTESIAN_POINT('Ctrl Pts',(0.000250354759005367,19.822070567486,
-20.4060840648359));
#22690=CARTESIAN_POINT('Ctrl Pts',(0.000214259287211671,19.8201408744217,
-20.4041086829836));
#22691=CARTESIAN_POINT('Ctrl Pts',(0.000181286595136419,19.818165831286,
-20.4020864313805));
#22692=CARTESIAN_POINT('Ctrl Pts',(0.000152582218496233,19.8162007777884,
-20.4000741270848));
#22693=CARTESIAN_POINT('Ctrl Pts',(0.000112831070522241,19.8134794808468,
-20.3972873950533));
#22694=CARTESIAN_POINT('Ctrl Pts',(8.15437448740462E-5,19.810780228473,
-20.3945226994929));
#22695=CARTESIAN_POINT('Ctrl Pts',(5.91223029096088E-5,19.8083150148832,
-20.3919974420402));
#22696=CARTESIAN_POINT('Ctrl Pts',(4.23062214362809E-5,19.8064661046908,
-20.3901034989507));
#22697=CARTESIAN_POINT('Ctrl Pts',(3.03587444767948E-5,19.8047514794406,
-20.3883469399828));
#22698=CARTESIAN_POINT('Ctrl Pts',(2.20012425220517E-5,19.8032453943865,
-20.386803894467));
#22699=CARTESIAN_POINT('Ctrl Pts',(1.49980715364258E-5,19.8019833700149,
-20.3855108990666));
#22700=CARTESIAN_POINT('Ctrl Pts',(1.04703182236286E-5,19.8008681397575,
-20.3843681978484));
#22701=CARTESIAN_POINT('Ctrl Pts',(7.40902886198214E-6,19.7999176631319,
-20.3833942117421));
#22702=CARTESIAN_POINT('Ctrl Pts',(4.53081936859977E-6,19.7990240295926,
-20.3824784747024));
#22703=CARTESIAN_POINT('Ctrl Pts',(2.93234049434048E-6,19.7982764424602,
-20.3817122953783));
#22704=CARTESIAN_POINT('Ctrl Pts',(1.92044015556725E-6,19.7976595188611,
-20.3810799307538));
#22705=CARTESIAN_POINT('Ctrl Pts',(9.7728613478454E-7,19.7970845077156,
-20.3804905276126));
#22706=CARTESIAN_POINT('Ctrl Pts',(5.43064674007645E-7,19.7966231564816,
-20.3800175251989));
#22707=CARTESIAN_POINT('Ctrl Pts',(2.92653819400357E-7,19.7962322344865,
-20.3796166523707));
#22708=CARTESIAN_POINT('Ctrl Pts',(7.44390397725664E-8,19.7958915745054,
-20.3792673209648));
#22709=CARTESIAN_POINT('Ctrl Pts',(-2.22066279043125E-16,19.7956041314054,
-20.3789724910909));
#22710=CARTESIAN_POINT('Ctrl Pts',(-2.22044604925031E-16,19.7953186364093,
-20.3786796564404));
#22711=CARTESIAN_POINT('',(0.,20.1476593182046,-20.026338974645));
#22712=CARTESIAN_POINT('Ctrl Pts',(0.00185295431591431,19.8682455202995,
-20.4532144101331));
#22713=CARTESIAN_POINT('Ctrl Pts',(0.0210291123338008,20.2475554365488,
-20.8386547994645));
#22714=CARTESIAN_POINT('Ctrl Pts',(0.19417406045939,20.6353433627736,-21.1941740604579));
#22715=CARTESIAN_POINT('Ctrl Pts',(0.439339828216959,20.9273329823489,-21.439339828217));
#22716=CARTESIAN_POINT('Ctrl Pts',(0.00185295431591403,20.1036752647639,
-20.2177846656687));
#22717=CARTESIAN_POINT('Ctrl Pts',(0.0210291123338009,20.4850286720406,
-20.6011815639727));
#22718=CARTESIAN_POINT('Ctrl Pts',(0.194174060459389,20.8620603765216,-20.9674570467099));
#22719=CARTESIAN_POINT('Ctrl Pts',(0.439339828216958,21.1384420454914,-21.2282307650744));
#22720=CARTESIAN_POINT('Ctrl Pts',(0.00185295431591376,20.3391050092284,
-19.9823549212043));
#22721=CARTESIAN_POINT('Ctrl Pts',(0.021029112333801,20.7225019075324,-20.3637083284809));
#22722=CARTESIAN_POINT('Ctrl Pts',(0.194174060459389,21.0887773902696,-20.740740032962));
#22723=CARTESIAN_POINT('Ctrl Pts',(0.439339828216957,21.349551108634,-21.0171217019318));
#22724=CARTESIAN_POINT('Ctrl Pts',(0.00185295431591348,20.5745347536928,
-19.7469251767398));
#22725=CARTESIAN_POINT('Ctrl Pts',(0.0210291123338011,20.9599751430241,
-20.1262350929892));
#22726=CARTESIAN_POINT('Ctrl Pts',(0.194174060459389,21.3154944040175,-20.514023019214));
#22727=CARTESIAN_POINT('Ctrl Pts',(0.439339828216956,21.5606601717766,-20.8060126387892));
#22728=CARTESIAN_POINT('',(0.439339828216882,21.5606601717765,-20.8060126387891));
#22729=CARTESIAN_POINT('Ctrl Pts',(0.00185295431591348,20.5745347536928,
-19.7469251767398));
#22730=CARTESIAN_POINT('Ctrl Pts',(0.0210291123338011,20.9599751430241,
-20.1262350929892));
#22731=CARTESIAN_POINT('Ctrl Pts',(0.194174060459389,21.3154944040175,-20.514023019214));
#22732=CARTESIAN_POINT('Ctrl Pts',(0.439339828216956,21.5606601717766,-20.8060126387892));
#22733=CARTESIAN_POINT('',(0.439339828217853,20.9273329823471,-21.4393398282178));
#22734=CARTESIAN_POINT('',(0.439339828216882,21.5606601717765,-20.8060126387891));
#22735=CARTESIAN_POINT('Ctrl Pts',(0.439339828216959,20.9273329823489,-21.439339828217));
#22736=CARTESIAN_POINT('Ctrl Pts',(0.19417406045939,20.6353433627736,-21.1941740604579));
#22737=CARTESIAN_POINT('Ctrl Pts',(0.0210291123338008,20.2475554365488,
-20.8386547994645));
#22738=CARTESIAN_POINT('Ctrl Pts',(0.00185295431591431,19.8682455202995,
-20.4532144101331));
#22739=CARTESIAN_POINT('Ctrl Pts',(1.49999999999999,22.,-21.7953186364092));
#22740=CARTESIAN_POINT('Ctrl Pts',(1.21626217779757,22.,-21.5192990451721));
#22741=CARTESIAN_POINT('Ctrl Pts',(0.921462981006754,21.9185839147642,-21.2520540356058));
#22742=CARTESIAN_POINT('Ctrl Pts',(0.662909388853527,21.7447004895678,-21.0317299497988));
#22743=CARTESIAN_POINT('Ctrl Pts',(1.40374142648193,21.8220460536244,-21.9339538507548));
#22744=CARTESIAN_POINT('Ctrl Pts',(1.1406737996242,21.8044458905108,-21.6760317112072));
#22745=CARTESIAN_POINT('Ctrl Pts',(0.877124322932673,21.7115209147256,-21.4308516926654));
#22746=CARTESIAN_POINT('Ctrl Pts',(0.65642758371972,21.5472709534839,-21.2356412910166));
#22747=CARTESIAN_POINT('Ctrl Pts',(1.30748285296387,21.6440921072489,-22.0725890651003));
#22748=CARTESIAN_POINT('Ctrl Pts',(1.06508542145083,21.6088917810216,-21.8327643772423));
#22749=CARTESIAN_POINT('Ctrl Pts',(0.832785664858593,21.504457914687,-21.6096493497249));
#22750=CARTESIAN_POINT('Ctrl Pts',(0.649945778585914,21.3498414173999,-21.4395526322343));
#22751=CARTESIAN_POINT('Ctrl Pts',(1.21122427944581,21.4661381608733,-22.2112242794458));
#22752=CARTESIAN_POINT('Ctrl Pts',(0.989497043277452,21.4133376715324,-21.9894970432775));
#22753=CARTESIAN_POINT('Ctrl Pts',(0.788447006784511,21.2973949146484,-21.7884470067845));
#22754=CARTESIAN_POINT('Ctrl Pts',(0.643463973452107,21.152411881316,-21.6434639734521));
#22755=CARTESIAN_POINT('',(1.49999999999999,22.,-21.7953186364092));
#22756=CARTESIAN_POINT('',(1.21122427944581,21.4661381608733,-22.2112242794458));
#22757=CARTESIAN_POINT('',(1.49999999999999,22.,-21.7953186364092));
#22758=CARTESIAN_POINT('',(0.643463973452109,21.152411881316,-21.6434639734521));
#22759=CARTESIAN_POINT('Ctrl Pts',(1.21122427944581,21.4661381608733,-22.2112242794458));
#22760=CARTESIAN_POINT('Ctrl Pts',(0.989497043277452,21.4133376715324,-21.9894970432775));
#22761=CARTESIAN_POINT('Ctrl Pts',(0.788447006784511,21.2973949146484,-21.7884470067845));
#22762=CARTESIAN_POINT('Ctrl Pts',(0.643463973452107,21.152411881316,-21.6434639734521));
#22763=CARTESIAN_POINT('',(0.662909388853531,21.7447004895678,-21.0317299497988));
#22764=CARTESIAN_POINT('',(0.643463973452109,21.152411881316,-21.6434639734521));
#22765=CARTESIAN_POINT('Ctrl Pts',(0.662909388853527,21.7447004895678,-21.0317299497988));
#22766=CARTESIAN_POINT('Ctrl Pts',(0.921462981006754,21.9185839147642,-21.2520540356058));
#22767=CARTESIAN_POINT('Ctrl Pts',(1.21626217779757,22.,-21.5192990451721));
#22768=CARTESIAN_POINT('Ctrl Pts',(1.49999999999999,22.,-21.7953186364092));
#22769=CARTESIAN_POINT('Ctrl Pts',(0.43933982821688,20.9273329823488,-21.4393398282169));
#22770=CARTESIAN_POINT('Ctrl Pts',(0.509453252888523,21.0108372675684,-21.5094532528885));
#22771=CARTESIAN_POINT('Ctrl Pts',(0.576934137750669,21.0858820456145,-21.5769341377507));
#22772=CARTESIAN_POINT('Ctrl Pts',(0.643463973452108,21.152411881316,-21.6434639734521));
#22773=CARTESIAN_POINT('Ctrl Pts',(0.43933982821688,21.1384420454913,-21.2282307650743));
#22774=CARTESIAN_POINT('Ctrl Pts',(0.509453252888438,21.2174827105284,-21.3028078099286));
#22775=CARTESIAN_POINT('Ctrl Pts',(0.579610088542197,21.2880143685876,-21.3730586867583));
#22776=CARTESIAN_POINT('Ctrl Pts',(0.649945778585916,21.3498414173999,-21.4395526322343));
#22777=CARTESIAN_POINT('Ctrl Pts',(0.439339828216881,21.3495511086339,-21.0171217019317));
#22778=CARTESIAN_POINT('Ctrl Pts',(0.509453252888354,21.4241281534884,-21.0961623669687));
#22779=CARTESIAN_POINT('Ctrl Pts',(0.582286039333725,21.4901466915607,-21.169183235766));
#22780=CARTESIAN_POINT('Ctrl Pts',(0.656427583719724,21.5472709534839,-21.2356412910166));
#22781=CARTESIAN_POINT('Ctrl Pts',(0.439339828216881,21.5606601717765,-20.8060126387891));
#22782=CARTESIAN_POINT('Ctrl Pts',(0.509453252888269,21.6307735964483,-20.8895169240087));
#22783=CARTESIAN_POINT('Ctrl Pts',(0.584961990125253,21.6922790145338,-20.9653077847737));
#22784=CARTESIAN_POINT('Ctrl Pts',(0.662909388853532,21.7447004895678,-21.0317299497988));
#22785=CARTESIAN_POINT('Ctrl Pts',(0.643463973452108,21.152411881316,-21.6434639734521));
#22786=CARTESIAN_POINT('Ctrl Pts',(0.576934137750669,21.0858820456145,-21.5769341377507));
#22787=CARTESIAN_POINT('Ctrl Pts',(0.509453252888523,21.0108372675684,-21.5094532528885));
#22788=CARTESIAN_POINT('Ctrl Pts',(0.43933982821688,20.9273329823488,-21.4393398282169));
#22789=CARTESIAN_POINT('Ctrl Pts',(0.439339828216881,21.5606601717765,-20.8060126387891));
#22790=CARTESIAN_POINT('Ctrl Pts',(0.509453252888269,21.6307735964483,-20.8895169240087));
#22791=CARTESIAN_POINT('Ctrl Pts',(0.584961990125253,21.6922790145338,-20.9653077847737));
#22792=CARTESIAN_POINT('Ctrl Pts',(0.662909388853532,21.7447004895678,-21.0317299497988));
#22793=CARTESIAN_POINT('Origin',(5.30177669529664,21.75,-25.9482233047034));
#22794=CARTESIAN_POINT('',(1.5,21.5,-22.5));
#22795=CARTESIAN_POINT('',(1.85355339059327,22.,-22.1464466094067));
#22796=CARTESIAN_POINT('',(1.5,21.5,-22.5));
#22797=CARTESIAN_POINT('',(2.85355339059327,22.,-23.1464466094067));
#22798=CARTESIAN_POINT('',(5.47855339059327,22.,-25.7714466094067));
#22799=CARTESIAN_POINT('',(2.5,21.5,-23.5));
#22800=CARTESIAN_POINT('',(2.85355339059327,22.,-23.1464466094067));
#22801=CARTESIAN_POINT('',(5.12500000000001,21.5,-26.125));
#22802=CARTESIAN_POINT('Ctrl Pts',(1.21122427944581,21.4661381608733,-22.2112242794458));
#22803=CARTESIAN_POINT('Ctrl Pts',(1.30519315757561,21.4885152167272,-22.3051931575756));
#22804=CARTESIAN_POINT('Ctrl Pts',(1.40259226494897,21.5,-22.402592264949));
#22805=CARTESIAN_POINT('Ctrl Pts',(1.5,21.5,-22.5));
#22806=CARTESIAN_POINT('Ctrl Pts',(1.30748285296387,21.6440921072489,-22.0725890651003));
#22807=CARTESIAN_POINT('Ctrl Pts',(1.4102118414925,21.6590101444848,-22.17422771471));
#22808=CARTESIAN_POINT('Ctrl Pts',(1.51394954614333,21.6666666666667,-22.2782472857478));
#22809=CARTESIAN_POINT('Ctrl Pts',(1.61785113019775,21.6666666666667,-22.3821488698022));
#22810=CARTESIAN_POINT('Ctrl Pts',(1.40374142648192,21.8220460536244,-21.9339538507548));
#22811=CARTESIAN_POINT('Ctrl Pts',(1.5152305254094,21.8295050722424,-22.0432622718444));
#22812=CARTESIAN_POINT('Ctrl Pts',(1.62530682733768,21.8333333333333,-22.1539023065467));
#22813=CARTESIAN_POINT('Ctrl Pts',(1.73570226039551,21.8333333333333,-22.2642977396045));
#22814=CARTESIAN_POINT('Ctrl Pts',(1.49999999999998,22.,-21.7953186364092));
#22815=CARTESIAN_POINT('Ctrl Pts',(1.62024920932629,22.,-21.9122968289787));
#22816=CARTESIAN_POINT('Ctrl Pts',(1.73666410853204,22.,-22.0295573273455));
#22817=CARTESIAN_POINT('Ctrl Pts',(1.85355339059327,22.,-22.1464466094067));
#22818=CARTESIAN_POINT('Ctrl Pts',(1.5,21.5,-22.5));
#22819=CARTESIAN_POINT('Ctrl Pts',(1.40259226494897,21.5,-22.402592264949));
#22820=CARTESIAN_POINT('Ctrl Pts',(1.30519315757561,21.4885152167272,-22.3051931575756));
#22821=CARTESIAN_POINT('Ctrl Pts',(1.21122427944581,21.4661381608733,-22.2112242794458));
#22822=CARTESIAN_POINT('Ctrl Pts',(1.49999999999998,22.,-21.7953186364092));
#22823=CARTESIAN_POINT('Ctrl Pts',(1.62024920932629,22.,-21.9122968289787));
#22824=CARTESIAN_POINT('Ctrl Pts',(1.73666410853204,22.,-22.0295573273455));
#22825=CARTESIAN_POINT('Ctrl Pts',(1.85355339059327,22.,-22.1464466094067));
#22826=CARTESIAN_POINT('Ctrl Pts',(3.96827005020121,21.7447004895678,-24.3370906111465));
#22827=CARTESIAN_POINT('Ctrl Pts',(3.74794596439424,21.9185839147642,-24.0785370189932));
#22828=CARTESIAN_POINT('Ctrl Pts',(3.48070095482788,22.,-23.7837378222024));
#22829=CARTESIAN_POINT('Ctrl Pts',(3.20468136359074,22.,-23.5));
#22830=CARTESIAN_POINT('Ctrl Pts',(3.76435870898344,21.5472709534839,-24.3435724162803));
#22831=CARTESIAN_POINT('Ctrl Pts',(3.56914830733465,21.7115209147256,-24.1228756770673));
#22832=CARTESIAN_POINT('Ctrl Pts',(3.32396828879277,21.8044458905108,-23.8593262003758));
#22833=CARTESIAN_POINT('Ctrl Pts',(3.06604614924522,21.8220460536244,-23.5962585735181));
#22834=CARTESIAN_POINT('Ctrl Pts',(3.56044736776567,21.3498414173999,-24.3500542214141));
#22835=CARTESIAN_POINT('Ctrl Pts',(3.39035065027507,21.504457914687,-24.1672143351414));
#22836=CARTESIAN_POINT('Ctrl Pts',(3.16723562275766,21.6088917810216,-23.9349145785492));
#22837=CARTESIAN_POINT('Ctrl Pts',(2.9274109348997,21.6440921072489,-23.6925171470361));
#22838=CARTESIAN_POINT('Ctrl Pts',(3.35653602654789,21.152411881316,-24.3565360265479));
#22839=CARTESIAN_POINT('Ctrl Pts',(3.21155299321549,21.2973949146484,-24.2115529932155));
#22840=CARTESIAN_POINT('Ctrl Pts',(3.01050295672254,21.4133376715324,-24.0105029567225));
#22841=CARTESIAN_POINT('Ctrl Pts',(2.78877572055418,21.4661381608733,-23.7887757205542));
#22842=CARTESIAN_POINT('',(2.78877572055418,21.4661381608733,-23.7887757205542));
#22843=CARTESIAN_POINT('',(3.20468136359075,22.,-23.5));
#22844=CARTESIAN_POINT('',(2.78877572055418,21.4661381608733,-23.7887757205542));
#22845=CARTESIAN_POINT('',(3.96827005020121,21.7447004895678,-24.3370906111465));
#22846=CARTESIAN_POINT('Ctrl Pts',(3.20468136359074,22.,-23.5));
#22847=CARTESIAN_POINT('Ctrl Pts',(3.48070095482788,22.,-23.7837378222024));
#22848=CARTESIAN_POINT('Ctrl Pts',(3.74794596439424,21.9185839147642,-24.0785370189932));
#22849=CARTESIAN_POINT('Ctrl Pts',(3.96827005020121,21.7447004895678,-24.3370906111465));
#22850=CARTESIAN_POINT('',(3.35653602654789,21.152411881316,-24.3565360265479));
#22851=CARTESIAN_POINT('',(3.96827005020121,21.7447004895678,-24.3370906111465));
#22852=CARTESIAN_POINT('Ctrl Pts',(3.35653602654789,21.152411881316,-24.3565360265479));
#22853=CARTESIAN_POINT('Ctrl Pts',(3.21155299321549,21.2973949146484,-24.2115529932155));
#22854=CARTESIAN_POINT('Ctrl Pts',(3.01050295672254,21.4133376715324,-24.0105029567225));
#22855=CARTESIAN_POINT('Ctrl Pts',(2.78877572055418,21.4661381608733,-23.7887757205542));
#22856=CARTESIAN_POINT('Ctrl Pts',(2.5,21.5,-23.5));
#22857=CARTESIAN_POINT('Ctrl Pts',(2.59740773505102,21.5,-23.597407735051));
#22858=CARTESIAN_POINT('Ctrl Pts',(2.69480684242438,21.4885152167272,-23.6948068424244));
#22859=CARTESIAN_POINT('Ctrl Pts',(2.78877572055418,21.4661381608733,-23.7887757205542));
#22860=CARTESIAN_POINT('Ctrl Pts',(2.61785113019776,21.6666666666667,-23.3821488698022));
#22861=CARTESIAN_POINT('Ctrl Pts',(2.72175271425219,21.6666666666667,-23.4860504538567));
#22862=CARTESIAN_POINT('Ctrl Pts',(2.82577228529002,21.6590101444848,-23.5897881585075));
#22863=CARTESIAN_POINT('Ctrl Pts',(2.92741093489971,21.6440921072489,-23.6925171470361));
#22864=CARTESIAN_POINT('Ctrl Pts',(2.73570226039552,21.8333333333333,-23.2642977396045));
#22865=CARTESIAN_POINT('Ctrl Pts',(2.84609769345335,21.8333333333333,-23.3746931726623));
#22866=CARTESIAN_POINT('Ctrl Pts',(2.95673772815565,21.8295050722424,-23.4847694745906));
#22867=CARTESIAN_POINT('Ctrl Pts',(3.06604614924523,21.8220460536244,-23.5962585735181));
#22868=CARTESIAN_POINT('Ctrl Pts',(2.85355339059328,22.,-23.1464466094067));
#22869=CARTESIAN_POINT('Ctrl Pts',(2.97044267265451,22.,-23.263335891468));
#22870=CARTESIAN_POINT('Ctrl Pts',(3.08770317102128,22.,-23.3797507906737));
#22871=CARTESIAN_POINT('Ctrl Pts',(3.20468136359075,22.,-23.5));
#22872=CARTESIAN_POINT('Ctrl Pts',(2.78877572055418,21.4661381608733,-23.7887757205542));
#22873=CARTESIAN_POINT('Ctrl Pts',(2.69480684242438,21.4885152167272,-23.6948068424244));
#22874=CARTESIAN_POINT('Ctrl Pts',(2.59740773505102,21.5,-23.597407735051));
#22875=CARTESIAN_POINT('Ctrl Pts',(2.5,21.5,-23.5));
#22876=CARTESIAN_POINT('Ctrl Pts',(2.85355339059328,22.,-23.1464466094067));
#22877=CARTESIAN_POINT('Ctrl Pts',(2.97044267265451,22.,-23.263335891468));
#22878=CARTESIAN_POINT('Ctrl Pts',(3.08770317102128,22.,-23.3797507906737));
#22879=CARTESIAN_POINT('Ctrl Pts',(3.20468136359075,22.,-23.5));
#22880=CARTESIAN_POINT('Ctrl Pts',(3.56066017178304,20.9273329823489,-24.560660171783));
#22881=CARTESIAN_POINT('Ctrl Pts',(3.8058259395421,20.6353433627736,-24.8058259395406));
#22882=CARTESIAN_POINT('Ctrl Pts',(4.16134520053552,20.2475554365488,-24.9789708876662));
#22883=CARTESIAN_POINT('Ctrl Pts',(4.54678558986685,19.8682455202995,-24.9981470456841));
#22884=CARTESIAN_POINT('Ctrl Pts',(3.77176923492562,21.1384420454914,-24.560660171783));
#22885=CARTESIAN_POINT('Ctrl Pts',(4.03254295329006,20.8620603765216,-24.8058259395406));
#22886=CARTESIAN_POINT('Ctrl Pts',(4.39881843602729,20.4850286720406,-24.9789708876662));
#22887=CARTESIAN_POINT('Ctrl Pts',(4.7822153343313,20.1036752647639,-24.9981470456841));
#22888=CARTESIAN_POINT('Ctrl Pts',(3.9828782980682,21.349551108634,-24.560660171783));
#22889=CARTESIAN_POINT('Ctrl Pts',(4.25925996703803,21.0887773902696,-24.8058259395406));
#22890=CARTESIAN_POINT('Ctrl Pts',(4.63629167151906,20.7225019075324,-24.9789708876662));
#22891=CARTESIAN_POINT('Ctrl Pts',(5.01764507879574,20.3391050092283,-24.9981470456841));
#22892=CARTESIAN_POINT('Ctrl Pts',(4.19398736121078,21.5606601717766,-24.560660171783));
#22893=CARTESIAN_POINT('Ctrl Pts',(4.48597698078599,21.3154944040175,-24.8058259395406));
#22894=CARTESIAN_POINT('Ctrl Pts',(4.87376490701083,20.9599751430241,-24.9789708876662));
#22895=CARTESIAN_POINT('Ctrl Pts',(5.25307482326019,20.5745347536928,-24.9981470456841));
#22896=CARTESIAN_POINT('',(3.56066017178215,20.9273329823471,-24.5606601717821));
#22897=CARTESIAN_POINT('Ctrl Pts',(4.54678558986685,19.8682455202995,-24.9981470456841));
#22898=CARTESIAN_POINT('Ctrl Pts',(4.16134520053552,20.2475554365488,-24.9789708876662));
#22899=CARTESIAN_POINT('Ctrl Pts',(3.8058259395421,20.6353433627736,-24.8058259395406));
#22900=CARTESIAN_POINT('Ctrl Pts',(3.56066017178304,20.9273329823489,-24.560660171783));
#22901=CARTESIAN_POINT('',(4.19398736121088,21.5606601717765,-24.5606601717831));
#22902=CARTESIAN_POINT('',(3.56066017178215,20.9273329823471,-24.5606601717821));
#22903=CARTESIAN_POINT('Ctrl Pts',(4.19398736121078,21.5606601717766,-24.560660171783));
#22904=CARTESIAN_POINT('Ctrl Pts',(4.48597698078599,21.3154944040175,-24.8058259395406));
#22905=CARTESIAN_POINT('Ctrl Pts',(4.87376490701083,20.9599751430241,-24.9789708876662));
#22906=CARTESIAN_POINT('Ctrl Pts',(5.25307482326019,20.5745347536928,-24.9981470456841));
#22907=CARTESIAN_POINT('Ctrl Pts',(3.35653602654789,21.1524118813159,-24.3565360265479));
#22908=CARTESIAN_POINT('Ctrl Pts',(3.42306586224933,21.0858820456145,-24.4230658622493));
#22909=CARTESIAN_POINT('Ctrl Pts',(3.49054674711148,21.0108372675684,-24.4905467471115));
#22910=CARTESIAN_POINT('Ctrl Pts',(3.56066017178311,20.9273329823488,-24.5606601717831));
#22911=CARTESIAN_POINT('Ctrl Pts',(3.56044736776567,21.3498414173999,-24.3500542214141));
#22912=CARTESIAN_POINT('Ctrl Pts',(3.62694131324166,21.2880143685876,-24.4203899114578));
#22913=CARTESIAN_POINT('Ctrl Pts',(3.6971921900714,21.2174827105284,-24.4905467471116));
#22914=CARTESIAN_POINT('Ctrl Pts',(3.7717692349257,21.1384420454914,-24.5606601717831));
#22915=CARTESIAN_POINT('Ctrl Pts',(3.76435870898344,21.5472709534839,-24.3435724162803));
#22916=CARTESIAN_POINT('Ctrl Pts',(3.830816764234,21.4901466915607,-24.4177139606663));
#22917=CARTESIAN_POINT('Ctrl Pts',(3.90383763303133,21.4241281534884,-24.4905467471116));
#22918=CARTESIAN_POINT('Ctrl Pts',(3.98287829806829,21.3495511086339,-24.5606601717831));
#22919=CARTESIAN_POINT('Ctrl Pts',(3.96827005020121,21.7447004895678,-24.3370906111465));
#22920=CARTESIAN_POINT('Ctrl Pts',(4.03469221522633,21.6922790145338,-24.4150380098747));
#22921=CARTESIAN_POINT('Ctrl Pts',(4.11048307599125,21.6307735964483,-24.4905467471117));
#22922=CARTESIAN_POINT('Ctrl Pts',(4.19398736121087,21.5606601717765,-24.5606601717831));
#22923=CARTESIAN_POINT('Ctrl Pts',(3.56066017178311,20.9273329823488,-24.5606601717831));
#22924=CARTESIAN_POINT('Ctrl Pts',(3.49054674711148,21.0108372675684,-24.4905467471115));
#22925=CARTESIAN_POINT('Ctrl Pts',(3.42306586224933,21.0858820456145,-24.4230658622493));
#22926=CARTESIAN_POINT('Ctrl Pts',(3.35653602654789,21.1524118813159,-24.3565360265479));
#22927=CARTESIAN_POINT('Ctrl Pts',(3.96827005020121,21.7447004895678,-24.3370906111465));
#22928=CARTESIAN_POINT('Ctrl Pts',(4.03469221522633,21.6922790145338,-24.4150380098747));
#22929=CARTESIAN_POINT('Ctrl Pts',(4.11048307599125,21.6307735964483,-24.4905467471117));
#22930=CARTESIAN_POINT('Ctrl Pts',(4.19398736121087,21.5606601717765,-24.5606601717831));
#22931=CARTESIAN_POINT('Origin',(1.5,20.5,-6.25));
#22932=CARTESIAN_POINT('',(0.,20.5,35.3786796564404));
#22933=CARTESIAN_POINT('',(0.,20.5,-6.25));
#22934=CARTESIAN_POINT('',(1.5,22.,35.3786796564404));
#22935=CARTESIAN_POINT('Origin',(1.5,20.5,35.3786796564404));
#22936=CARTESIAN_POINT('',(1.5,22.,-6.25));
#22937=CARTESIAN_POINT('Origin',(0.,-22.,-21.));
#22938=CARTESIAN_POINT('',(0.,-20.5,-20.3786796564404));
#22939=CARTESIAN_POINT('',(0.,-22.,-20.3786796564404));
#22940=CARTESIAN_POINT('',(0.,-20.5,35.3786796564404));
#22941=CARTESIAN_POINT('',(0.,-20.5,-6.25));
#22942=CARTESIAN_POINT('',(0.,-22.,35.3786796564404));
#22943=CARTESIAN_POINT('Origin',(1.5,-22.,-20.3786796564404));
#22944=CARTESIAN_POINT('',(0.439339828220176,-20.5,-21.4393398282202));
#22945=CARTESIAN_POINT('',(0.439339828220176,-22.,-21.4393398282202));
#22946=CARTESIAN_POINT('Origin',(1.5,-20.5,-20.3786796564404));
#22947=CARTESIAN_POINT('Origin',(4.,-22.,-25.));
#22948=CARTESIAN_POINT('',(3.56066017177982,-20.5,-24.5606601717798));
#22949=CARTESIAN_POINT('',(3.56066017177982,-22.,-24.5606601717798));
#22950=CARTESIAN_POINT('',(5.125,-20.5,-26.125));
#22951=CARTESIAN_POINT('Origin',(56.,-20.5,-23.5));
#22952=CARTESIAN_POINT('',(61.5,-22.,-23.5));
#22953=CARTESIAN_POINT('',(61.5,-20.5,-25.));
#22954=CARTESIAN_POINT('Origin',(61.5,-20.5,-23.5));
#22955=CARTESIAN_POINT('',(68.5,-20.5,-25.));
#22956=CARTESIAN_POINT('',(56.,-20.5,-25.));
#22957=CARTESIAN_POINT('',(68.5,-22.,-23.5));
#22958=CARTESIAN_POINT('Origin',(68.5,-20.5,-23.5));
#22959=CARTESIAN_POINT('',(56.,-22.,-23.5));
#22960=CARTESIAN_POINT('Origin',(68.5,-20.5,-23.5));
#22961=CARTESIAN_POINT('',(70.,-20.5,-23.5));
#22962=CARTESIAN_POINT('Origin',(68.5,-20.5,-23.5));
#22963=CARTESIAN_POINT('Origin',(68.5,-20.5,-23.5));
#22964=CARTESIAN_POINT('Origin',(61.5,-20.5,-23.5));
#22965=CARTESIAN_POINT('Origin',(61.5,-20.5,-23.5));
#22966=CARTESIAN_POINT('Origin',(61.5,-20.5,-23.5));
#22967=CARTESIAN_POINT('Origin',(68.5,-20.5,4.25));
#22968=CARTESIAN_POINT('',(70.,-20.5,-17.5712833908056));
#22969=CARTESIAN_POINT('',(70.,-20.5,4.25));
#22970=CARTESIAN_POINT('',(68.5,-22.,-15.6524758424985));
#22971=CARTESIAN_POINT('Ctrl Pts',(68.5,-22.,-15.6524758424985));
#22972=CARTESIAN_POINT('Ctrl Pts',(68.5946178513885,-22.,-15.6524758424985));
#22973=CARTESIAN_POINT('Ctrl Pts',(68.6889643978921,-21.9909261474626,-15.665250854624));
#22974=CARTESIAN_POINT('Ctrl Pts',(68.8710686191993,-21.9563375109926,-15.7136914161295));
#22975=CARTESIAN_POINT('Ctrl Pts',(68.9588244922017,-21.9308152339295,-15.7493583883479));
#22976=CARTESIAN_POINT('Ctrl Pts',(69.2051881089356,-21.8355590404292,-15.88144036437));
#22977=CARTESIAN_POINT('Ctrl Pts',(69.3468785813891,-21.7463710185311,-16.0037159774975));
#22978=CARTESIAN_POINT('Ctrl Pts',(69.6391148171733,-21.5040391092436,-16.3291117577357));
#22979=CARTESIAN_POINT('Ctrl Pts',(69.7765132729404,-21.3178359703858,-16.572666547787));
#22980=CARTESIAN_POINT('Ctrl Pts',(69.9575260447372,-20.9170846786411,-17.0756837501162));
#22981=CARTESIAN_POINT('Ctrl Pts',(70.,-20.7022477383282,-17.3353257465337));
#22982=CARTESIAN_POINT('Ctrl Pts',(70.,-20.5,-17.5712833908056));
#22983=CARTESIAN_POINT('',(68.5,-22.,4.25));
#22984=CARTESIAN_POINT('Origin',(68.5,-22.,-23.5));
#22985=CARTESIAN_POINT('',(68.5,-10.1980390271856,-25.));
#22986=CARTESIAN_POINT('',(68.5,-22.,-25.));
#22987=CARTESIAN_POINT('',(70.,-13.2947358003083,-23.5));
#22988=CARTESIAN_POINT('Ctrl Pts',(70.,-13.2947358003083,-23.5));
#22989=CARTESIAN_POINT('Ctrl Pts',(70.,-12.5253526611459,-23.9352657686969));
#22990=CARTESIAN_POINT('Ctrl Pts',(69.8122976763679,-11.5896482415098,-24.3983540225569));
#22991=CARTESIAN_POINT('Ctrl Pts',(69.2682778073745,-10.6853817343331,-24.7965377420129));
#22992=CARTESIAN_POINT('Ctrl Pts',(69.099996626182,-10.4648018594106,-24.889928820497));
#22993=CARTESIAN_POINT('Ctrl Pts',(68.8470061948633,-10.2945164376804,-24.9604604345961));
#22994=CARTESIAN_POINT('Ctrl Pts',(68.7815873963742,-10.2591413018302,-24.97500159694));
#22995=CARTESIAN_POINT('Ctrl Pts',(68.64269539724,-10.2107026186997,-24.9948442089972));
#22996=CARTESIAN_POINT('Ctrl Pts',(68.5690622745619,-10.1980390271856,-25.));
#22997=CARTESIAN_POINT('Ctrl Pts',(68.5,-10.1980390271856,-25.));
#22998=CARTESIAN_POINT('',(70.,-22.,-23.5));
#22999=CARTESIAN_POINT('Origin',(70.,-22.,-25.));
#23000=CARTESIAN_POINT('',(61.5,-10.1980390271856,-25.));
#23001=CARTESIAN_POINT('',(61.5,-22.,-25.));
#23002=CARTESIAN_POINT('',(75.5,-10.1980390271856,-25.));
#23003=CARTESIAN_POINT('Origin',(82.5,20.5,21.2280731570623));
#23004=CARTESIAN_POINT('',(82.5,22.,21.2280731570623));
#23005=CARTESIAN_POINT('Origin',(82.5,20.5,21.2280731570623));
#23006=CARTESIAN_POINT('',(84.,20.5,21.2280731570623));
#23007=CARTESIAN_POINT('Origin',(82.5,20.5,21.2280731570623));
#23008=CARTESIAN_POINT('Origin',(82.5,20.5,21.2280731570623));
#23009=CARTESIAN_POINT('Origin',(82.5,-22.,21.2280731570623));
#23010=CARTESIAN_POINT('',(84.,16.6843912097029,21.2280731570623));
#23011=CARTESIAN_POINT('Ctrl Pts',(84.,16.6843912097029,21.2280731570623));
#23012=CARTESIAN_POINT('Ctrl Pts',(84.,16.424239791648,21.4325414571512));
#23013=CARTESIAN_POINT('Ctrl Pts',(83.9566902724278,16.1377744699131,21.6492625703158));
#23014=CARTESIAN_POINT('Ctrl Pts',(83.7720906996842,15.5809736161534,22.053380597491));
#23015=CARTESIAN_POINT('Ctrl Pts',(83.6323380105135,15.3103686972935,22.2411069388649));
#23016=CARTESIAN_POINT('Ctrl Pts',(83.4216450393869,15.0568236851315,22.4118978779271));
#23017=CARTESIAN_POINT('Ctrl Pts',(83.3973987301277,15.0292019594189,22.4304294784802));
#23018=CARTESIAN_POINT('Ctrl Pts',(83.3718572905786,15.0019020194829,22.4486733638724));
#23019=CARTESIAN_POINT('',(84.,-22.,21.2280731570623));
#23020=CARTESIAN_POINT('Origin',(82.5,20.5,15.25));
#23021=CARTESIAN_POINT('',(84.,20.5,17.5712833908056));
#23022=CARTESIAN_POINT('',(82.5,22.,15.6524758424985));
#23023=CARTESIAN_POINT('Ctrl Pts',(82.5,22.,15.6524758424985));
#23024=CARTESIAN_POINT('Ctrl Pts',(82.5946178513885,22.,15.6524758424985));
#23025=CARTESIAN_POINT('Ctrl Pts',(82.6889643978921,21.9909261474626,15.665250854624));
#23026=CARTESIAN_POINT('Ctrl Pts',(82.8710686191993,21.9563375109926,15.7136914161295));
#23027=CARTESIAN_POINT('Ctrl Pts',(82.9588244922017,21.9308152339295,15.7493583883479));
#23028=CARTESIAN_POINT('Ctrl Pts',(83.2051881089356,21.8355590404292,15.88144036437));
#23029=CARTESIAN_POINT('Ctrl Pts',(83.3468785813891,21.7463710185311,16.0037159774975));
#23030=CARTESIAN_POINT('Ctrl Pts',(83.6391148171733,21.5040391092436,16.3291117577357));
#23031=CARTESIAN_POINT('Ctrl Pts',(83.7765132729403,21.3178359703858,16.572666547787));
#23032=CARTESIAN_POINT('Ctrl Pts',(83.9575260447373,20.9170846786411,17.0756837501162));
#23033=CARTESIAN_POINT('Ctrl Pts',(84.,20.7022477383282,17.3353257465337));
#23034=CARTESIAN_POINT('Ctrl Pts',(84.,20.5,17.5712833908056));
#23035=CARTESIAN_POINT('',(82.5,22.,15.25));
#23036=CARTESIAN_POINT('',(84.,20.5,15.25));
#23037=CARTESIAN_POINT('Origin',(55.5193024198872,20.5,40.5));
#23038=CARTESIAN_POINT('',(55.5193024198872,20.5,42.));
#23039=CARTESIAN_POINT('',(55.5193024198872,22.,40.5));
#23040=CARTESIAN_POINT('Origin',(55.5193024198872,20.5,40.5));
#23041=CARTESIAN_POINT('Origin',(55.5193024198872,20.5,40.5));
#23042=CARTESIAN_POINT('Origin',(55.5193024198872,20.5,40.5));
#23043=CARTESIAN_POINT('Origin',(55.5193024198872,-20.5,40.5));
#23044=CARTESIAN_POINT('',(55.5193024198872,-20.5,42.));
#23045=CARTESIAN_POINT('Origin',(55.5193024198872,-20.5,40.5));
#23046=CARTESIAN_POINT('Origin',(55.5193024198872,-20.5,40.5));
#23047=CARTESIAN_POINT('Origin',(55.5193024198872,-22.,40.5));
#23048=CARTESIAN_POINT('',(55.5193024198872,-22.,42.));
#23049=CARTESIAN_POINT('Origin',(58.4153048715835,20.5,38.4314268202169));
#23050=CARTESIAN_POINT('',(58.4153048715835,22.,38.4314268202169));
#23051=CARTESIAN_POINT('Origin',(6.62132034355964,20.5,40.5));
#23052=CARTESIAN_POINT('',(5.56066017177982,20.5,41.5606601717798));
#23053=CARTESIAN_POINT('',(6.62132034355964,22.,40.5));
#23054=CARTESIAN_POINT('Origin',(6.62132034355965,20.5,40.5));
#23055=CARTESIAN_POINT('',(6.62132034355964,20.5,42.));
#23056=CARTESIAN_POINT('Origin',(6.62132034355964,20.5,40.5));
#23057=CARTESIAN_POINT('Origin',(6.62132034355964,20.5,40.5));
#23058=CARTESIAN_POINT('Origin',(6.62132034355964,-20.5,40.5));
#23059=CARTESIAN_POINT('',(6.62132034355964,-20.5,42.));
#23060=CARTESIAN_POINT('',(5.56066017177982,-20.5,41.5606601717798));
#23061=CARTESIAN_POINT('Origin',(6.62132034355964,-20.5,40.5));
#23062=CARTESIAN_POINT('Origin',(6.62132034355965,-20.5,40.5));
#23063=CARTESIAN_POINT('Origin',(6.62132034355964,-20.5,40.5));
#23064=CARTESIAN_POINT('Origin',(6.62132034355964,-22.,40.5));
#23065=CARTESIAN_POINT('',(6.62132034355964,-22.,42.));
#23066=CARTESIAN_POINT('',(5.56066017177982,-22.,41.5606601717798));
#23067=CARTESIAN_POINT('Origin',(24.,20.5,40.5));
#23068=CARTESIAN_POINT('',(24.,22.,40.5));
#23069=CARTESIAN_POINT('',(24.,20.5,42.));
#23070=CARTESIAN_POINT('Origin',(1.5,20.5,35.3786796564404));
#23071=CARTESIAN_POINT('',(0.439339828220176,20.5,36.4393398282202));
#23072=CARTESIAN_POINT('Origin',(1.5,20.5,35.3786796564404));
#23073=CARTESIAN_POINT('Origin',(1.5,20.5,35.3786796564404));
#23074=CARTESIAN_POINT('Origin',(1.5,-20.5,35.3786796564404));
#23075=CARTESIAN_POINT('',(0.439339828220176,-20.5,36.4393398282202));
#23076=CARTESIAN_POINT('Origin',(1.5,-20.5,35.3786796564404));
#23077=CARTESIAN_POINT('Origin',(1.5,-20.5,35.3786796564404));
#23078=CARTESIAN_POINT('Origin',(1.5,-20.5,35.3786796564404));
#23079=CARTESIAN_POINT('Origin',(1.5,-22.,35.3786796564404));
#23080=CARTESIAN_POINT('',(0.439339828220176,-22.,36.4393398282202));
#23081=CARTESIAN_POINT('Origin',(4.68566017177982,20.5,38.5643398282202));
#23082=CARTESIAN_POINT('',(4.68566017177982,22.,38.5643398282202));
#23083=CARTESIAN_POINT('',(3.625,20.5,39.625));
#23084=CARTESIAN_POINT('Origin',(4.62132034355965,-20.5,-23.5));
#23085=CARTESIAN_POINT('',(4.62132034355965,-20.5,-25.));
#23086=CARTESIAN_POINT('Origin',(4.62132034355965,-20.5,-23.5));
#23087=CARTESIAN_POINT('Origin',(4.62132034355965,-20.5,-23.5));
#23088=CARTESIAN_POINT('Origin',(4.62132034355964,-20.5,-23.5));
#23089=CARTESIAN_POINT('Origin',(56.,-20.5,-23.5));
#23090=CARTESIAN_POINT('',(13.5,-20.5,-25.));
#23091=CARTESIAN_POINT('Origin',(13.5,-20.5,-23.5));
#23092=CARTESIAN_POINT('',(56.,-20.5,-25.));
#23093=CARTESIAN_POINT('Origin',(13.5,-20.5,-23.5));
#23094=CARTESIAN_POINT('',(15.,-20.5,-23.5));
#23095=CARTESIAN_POINT('Origin',(13.5,-20.5,-23.5));
#23096=CARTESIAN_POINT('Origin',(13.5,-20.5,-23.5));
#23097=CARTESIAN_POINT('Origin',(6.18566017177982,-20.5,-25.0643398282202));
#23098=CARTESIAN_POINT('Origin',(1.5,-20.5,-20.3786796564404));
#23099=CARTESIAN_POINT('Origin',(4.62132034355965,-22.,-23.5));
#23100=CARTESIAN_POINT('',(4.62132034355965,-22.,-25.));
#23101=CARTESIAN_POINT('Origin',(13.5,20.5,-23.5));
#23102=CARTESIAN_POINT('',(13.5,20.5,-25.));
#23103=CARTESIAN_POINT('',(13.5,22.,-23.5));
#23104=CARTESIAN_POINT('Origin',(13.5,20.5,-23.5));
#23105=CARTESIAN_POINT('',(15.,20.5,-23.5));
#23106=CARTESIAN_POINT('Origin',(13.5,20.5,-23.5));
#23107=CARTESIAN_POINT('Origin',(13.5,20.5,-23.5));
#23108=CARTESIAN_POINT('Origin',(56.,20.5,-23.5));
#23109=CARTESIAN_POINT('',(56.,22.,-23.5));
#23110=CARTESIAN_POINT('',(56.,20.5,-25.));
#23111=CARTESIAN_POINT('Origin',(1.5,-20.5,-20.3786796564404));
#23112=CARTESIAN_POINT('Origin',(1.5,-20.5,-20.3786796564404));
#23113=CARTESIAN_POINT('Origin',(6.,-22.,42.));
#23114=CARTESIAN_POINT('',(24.,-20.5,42.));
#23115=CARTESIAN_POINT('',(32.5358115136623,-2.58526623249054,42.));
#23116=CARTESIAN_POINT('',(31.2738743424416,-2.24420189857483,42.));
#23117=CARTESIAN_POINT('Ctrl Pts',(32.5358115136623,-2.58526623249054,42.));
#23118=CARTESIAN_POINT('Ctrl Pts',(31.8298088014126,-2.58526623249054,42.));
#23119=CARTESIAN_POINT('Ctrl Pts',(31.2738743424416,-2.24420189857483,42.));
#23120=CARTESIAN_POINT('',(30.4314459860325,-1.31309688091278,42.));
#23121=CARTESIAN_POINT('Ctrl Pts',(31.2738743424416,-2.24420189857483,42.));
#23122=CARTESIAN_POINT('Ctrl Pts',(30.7179398834705,-1.90313756465912,42.));
#23123=CARTESIAN_POINT('Ctrl Pts',(30.4314459860325,-1.31309688091278,42.));
#23124=CARTESIAN_POINT('',(30.1449521258473,-0.0648021697998047,42.));
#23125=CARTESIAN_POINT('Ctrl Pts',(30.4314459860325,-1.31309688091278,42.));
#23126=CARTESIAN_POINT('Ctrl Pts',(30.1449521258473,-0.723056197166443,
42.));
#23127=CARTESIAN_POINT('Ctrl Pts',(30.1449521258473,-0.0648021697998047,
42.));
#23128=CARTESIAN_POINT('',(30.8134378492832,1.88437908887863,42.));
#23129=CARTESIAN_POINT('Ctrl Pts',(30.1449521258473,-0.0648021697998047,
42.));
#23130=CARTESIAN_POINT('Ctrl Pts',(30.1449521258473,1.1800816655159,42.));
#23131=CARTESIAN_POINT('Ctrl Pts',(30.8134378492832,1.88437908887863,42.));
#23132=CARTESIAN_POINT('',(32.5392223894596,2.58867621421814,42.));
#23133=CARTESIAN_POINT('Ctrl Pts',(30.8134378492832,1.88437908887863,42.));
#23134=CARTESIAN_POINT('Ctrl Pts',(31.4819234609604,2.58867621421814,42.));
#23135=CARTESIAN_POINT('Ctrl Pts',(32.5392223894596,2.58867621421814,42.));
#23136=CARTESIAN_POINT('',(33.7875168025494,2.25784420967102,42.));
#23137=CARTESIAN_POINT('Ctrl Pts',(32.5392223894596,2.58867621421814,42.));
#23138=CARTESIAN_POINT('Ctrl Pts',(33.23158249259,2.58867621421814,42.));
#23139=CARTESIAN_POINT('Ctrl Pts',(33.7875168025494,2.25784420967102,42.));
#23140=CARTESIAN_POINT('',(34.6350611746311,1.33526593446732,42.));
#23141=CARTESIAN_POINT('Ctrl Pts',(33.7875168025494,2.25784420967102,42.));
#23142=CARTESIAN_POINT('Ctrl Pts',(34.343451410532,1.92701190710068,42.));
#23143=CARTESIAN_POINT('Ctrl Pts',(34.6350611746311,1.33526593446732,42.));
#23144=CARTESIAN_POINT('',(34.9266712367535,-0.00682175159454346,42.));
#23145=CARTESIAN_POINT('Ctrl Pts',(34.6350611746311,1.33526593446732,42.));
#23146=CARTESIAN_POINT('Ctrl Pts',(34.9266712367535,0.74351966381073,42.));
#23147=CARTESIAN_POINT('Ctrl Pts',(34.9266712367535,-0.00682175159454346,
42.));
#23148=CARTESIAN_POINT('',(34.6197132766247,-1.36766731739044,42.));
#23149=CARTESIAN_POINT('Ctrl Pts',(34.9266712367535,-0.00682175159454346,
42.));
#23150=CARTESIAN_POINT('Ctrl Pts',(34.9266712367535,-0.767394304275513,
42.));
#23151=CARTESIAN_POINT('Ctrl Pts',(34.6197132766247,-1.36766731739044,42.));
#23152=CARTESIAN_POINT('',(33.7499998509884,-2.27660298347473,42.));
#23153=CARTESIAN_POINT('Ctrl Pts',(34.6197132766247,-1.36766731739044,42.));
#23154=CARTESIAN_POINT('Ctrl Pts',(34.3127556145191,-1.96793973445892,42.));
#23155=CARTESIAN_POINT('Ctrl Pts',(33.7499998509884,-2.27660298347473,42.));
#23156=CARTESIAN_POINT('Ctrl Pts',(33.7499998509884,-2.27660298347473,42.));
#23157=CARTESIAN_POINT('Ctrl Pts',(33.1872440874577,-2.58526623249054,42.));
#23158=CARTESIAN_POINT('Ctrl Pts',(32.5358115136623,-2.58526623249054,42.));
#23159=CARTESIAN_POINT('',(29.667462259531,1.90995901823044,42.));
#23160=CARTESIAN_POINT('',(28.0133013427258,1.90995901823044,42.));
#23161=CARTESIAN_POINT('',(17.8337311297655,1.90995901823044,42.));
#23162=CARTESIAN_POINT('',(28.0133013427258,-2.5,42.));
#23163=CARTESIAN_POINT('',(28.0133013427258,-10.0450204908848,42.));
#23164=CARTESIAN_POINT('',(27.3516370356083,-2.5,42.));
#23165=CARTESIAN_POINT('',(17.0066506713629,-2.5,42.));
#23166=CARTESIAN_POINT('',(27.3516370356083,1.90995901823044,42.));
#23167=CARTESIAN_POINT('',(27.3516370356083,-12.25,42.));
#23168=CARTESIAN_POINT('',(25.7042973488569,1.90995901823044,42.));
#23169=CARTESIAN_POINT('',(16.6758185178041,1.90995901823044,42.));
#23170=CARTESIAN_POINT('',(25.7042973488569,2.5,42.));
#23171=CARTESIAN_POINT('',(25.7042973488569,-10.0450204908848,42.));
#23172=CARTESIAN_POINT('',(29.667462259531,2.5,42.));
#23173=CARTESIAN_POINT('',(15.8521486744285,2.5,42.));
#23174=CARTESIAN_POINT('',(29.667462259531,-9.75,42.));
#23175=CARTESIAN_POINT('',(20.4519100487232,-2.14699864387512,42.));
#23176=CARTESIAN_POINT('',(19.9982947669923,-1.05388820171356,42.));
#23177=CARTESIAN_POINT('Ctrl Pts',(20.4519100487232,-2.14699864387512,42.));
#23178=CARTESIAN_POINT('Ctrl Pts',(19.9982947669923,-1.7087310552597,42.));
#23179=CARTESIAN_POINT('Ctrl Pts',(19.9982947669923,-1.05388820171356,42.));
#23180=CARTESIAN_POINT('',(20.2455662563443,-0.237039625644684,42.));
#23181=CARTESIAN_POINT('Ctrl Pts',(19.9982947669923,-1.05388820171356,42.));
#23182=CARTESIAN_POINT('Ctrl Pts',(19.9982947669923,-0.566166639328003,
42.));
#23183=CARTESIAN_POINT('Ctrl Pts',(20.2455662563443,-0.237039625644684,
42.));
#23184=CARTESIAN_POINT('',(20.94986371696,0.211459994316101,42.));
#23185=CARTESIAN_POINT('Ctrl Pts',(20.2455662563443,-0.237039625644684,
42.));
#23186=CARTESIAN_POINT('Ctrl Pts',(20.4928377270699,0.0920873880386353,
42.));
#23187=CARTESIAN_POINT('Ctrl Pts',(20.94986371696,0.211459994316101,42.));
#23188=CARTESIAN_POINT('',(20.3836972266436,0.610504746437073,42.));
#23189=CARTESIAN_POINT('Ctrl Pts',(20.94986371696,0.211459994316101,42.));
#23190=CARTESIAN_POINT('Ctrl Pts',(20.5678718537092,0.351296067237854,42.));
#23191=CARTESIAN_POINT('Ctrl Pts',(20.3836972266436,0.610504746437073,42.));
#23192=CARTESIAN_POINT('',(20.1995225995779,1.23124152421951,42.));
#23193=CARTESIAN_POINT('Ctrl Pts',(20.3836972266436,0.610504746437073,42.));
#23194=CARTESIAN_POINT('Ctrl Pts',(20.1995225995779,0.869713723659515,42.));
#23195=CARTESIAN_POINT('Ctrl Pts',(20.1995225995779,1.23124152421951,42.));
#23196=CARTESIAN_POINT('',(20.5917463451624,2.14870393276215,42.));
#23197=CARTESIAN_POINT('Ctrl Pts',(20.1995225995779,1.23124152421951,42.));
#23198=CARTESIAN_POINT('Ctrl Pts',(20.1995225995779,1.77694410085678,42.));
#23199=CARTESIAN_POINT('Ctrl Pts',(20.5917463451624,2.14870393276215,42.));
#23200=CARTESIAN_POINT('',(21.6354024410248,2.52046346664429,42.));
#23201=CARTESIAN_POINT('Ctrl Pts',(20.5917463451624,2.14870393276215,42.));
#23202=CARTESIAN_POINT('Ctrl Pts',(20.9839700162411,2.52046346664429,42.));
#23203=CARTESIAN_POINT('Ctrl Pts',(21.6354024410248,2.52046346664429,42.));
#23204=CARTESIAN_POINT('',(22.68929079175,2.14017748832703,42.));
#23205=CARTESIAN_POINT('Ctrl Pts',(21.6354024410248,2.52046346664429,42.));
#23206=CARTESIAN_POINT('Ctrl Pts',(22.2902457416058,2.52046346664429,42.));
#23207=CARTESIAN_POINT('Ctrl Pts',(22.68929079175,2.14017748832703,42.));
#23208=CARTESIAN_POINT('',(23.0883358418941,1.21418833732605,42.));
#23209=CARTESIAN_POINT('Ctrl Pts',(22.68929079175,2.14017748832703,42.));
#23210=CARTESIAN_POINT('Ctrl Pts',(23.0883358418941,1.75989091396332,42.));
#23211=CARTESIAN_POINT('Ctrl Pts',(23.0883358418941,1.21418833732605,42.));
#23212=CARTESIAN_POINT('',(22.9058663547039,0.608799457550049,42.));
#23213=CARTESIAN_POINT('Ctrl Pts',(23.0883358418941,1.21418833732605,42.));
#23214=CARTESIAN_POINT('Ctrl Pts',(23.0883358418941,0.866302847862244,42.));
#23215=CARTESIAN_POINT('Ctrl Pts',(22.9058663547039,0.608799457550049,42.));
#23216=CARTESIAN_POINT('',(22.3516373336315,0.211459994316101,42.));
#23217=CARTESIAN_POINT('Ctrl Pts',(22.9058663547039,0.608799457550049,42.));
#23218=CARTESIAN_POINT('Ctrl Pts',(22.7233971655369,0.351296067237854,42.));
#23219=CARTESIAN_POINT('Ctrl Pts',(22.3516373336315,0.211459994316101,42.));
#23220=CARTESIAN_POINT('',(23.0525241792202,-0.272851288318634,42.));
#23221=CARTESIAN_POINT('Ctrl Pts',(22.3516373336315,0.211459994316101,42.));
#23222=CARTESIAN_POINT('Ctrl Pts',(22.8120739758015,0.0613915920257568,
42.));
#23223=CARTESIAN_POINT('Ctrl Pts',(23.0525241792202,-0.272851288318634,
42.));
#23224=CARTESIAN_POINT('',(23.2929743826389,-1.07094138860703,42.));
#23225=CARTESIAN_POINT('Ctrl Pts',(23.0525241792202,-0.272851288318634,
42.));
#23226=CARTESIAN_POINT('Ctrl Pts',(23.2929743826389,-0.607094168663025,
42.));
#23227=CARTESIAN_POINT('Ctrl Pts',(23.2929743826389,-1.07094138860703,42.));
#23228=CARTESIAN_POINT('',(22.8393588960171,-2.14870393276215,42.));
#23229=CARTESIAN_POINT('Ctrl Pts',(23.2929743826389,-1.07094138860703,42.));
#23230=CARTESIAN_POINT('Ctrl Pts',(23.2929743826389,-1.71214163303375,42.));
#23231=CARTESIAN_POINT('Ctrl Pts',(22.8393588960171,-2.14870393276215,42.));
#23232=CARTESIAN_POINT('',(21.6456344723701,-2.58526623249054,42.));
#23233=CARTESIAN_POINT('Ctrl Pts',(22.8393588960171,-2.14870393276215,42.));
#23234=CARTESIAN_POINT('Ctrl Pts',(22.3857437074184,-2.58526623249054,42.));
#23235=CARTESIAN_POINT('Ctrl Pts',(21.6456344723701,-2.58526623249054,42.));
#23236=CARTESIAN_POINT('Ctrl Pts',(21.6456344723701,-2.58526623249054,42.));
#23237=CARTESIAN_POINT('Ctrl Pts',(20.9055253863335,-2.58526623249054,42.));
#23238=CARTESIAN_POINT('Ctrl Pts',(20.4519100487232,-2.14699864387512,42.));
#23239=CARTESIAN_POINT('',(39.0330834686756,-2.5,42.));
#23240=CARTESIAN_POINT('',(36.4068896323442,1.42905861139297,42.));
#23241=CARTESIAN_POINT('',(38.437241915911,-1.60855918115101,42.));
#23242=CARTESIAN_POINT('',(36.4068896323442,-2.5,42.));
#23243=CARTESIAN_POINT('',(36.4068896323442,-10.2854706943035,42.));
#23244=CARTESIAN_POINT('',(35.772510394454,-2.5,42.));
#23245=CARTESIAN_POINT('',(21.2034448161721,-2.5,42.));
#23246=CARTESIAN_POINT('',(35.772510394454,2.5,42.));
#23247=CARTESIAN_POINT('',(35.772510394454,-12.25,42.));
#23248=CARTESIAN_POINT('',(36.4512279629707,2.5,42.));
#23249=CARTESIAN_POINT('',(20.886255197227,2.5,42.));
#23250=CARTESIAN_POINT('',(39.0774215757847,-1.42564833164215,42.));
#23251=CARTESIAN_POINT('',(37.4052567618647,1.07391262226716,42.));
#23252=CARTESIAN_POINT('',(39.0774215757847,2.5,42.));
#23253=CARTESIAN_POINT('',(39.0774215757847,-11.7128241658211,42.));
#23254=CARTESIAN_POINT('',(39.7118009626865,2.5,42.));
#23255=CARTESIAN_POINT('',(22.5387107878923,2.5,42.));
#23256=CARTESIAN_POINT('',(39.7118009626865,-2.5,42.));
#23257=CARTESIAN_POINT('',(39.7118009626865,-9.75,42.));
#23258=CARTESIAN_POINT('',(22.8559004813433,-2.5,42.));
#23259=CARTESIAN_POINT('Origin',(0.,-22.,36.));
#23260=CARTESIAN_POINT('',(3.625,-20.5,39.625));
#23261=CARTESIAN_POINT('Origin',(4.68566017177982,-20.5,38.5643398282202));
#23262=CARTESIAN_POINT('Origin',(1.5,-20.5,-6.25));
#23263=CARTESIAN_POINT('Origin',(13.5,-20.5,-10.75));
#23264=CARTESIAN_POINT('',(15.,-20.5,18.));
#23265=CARTESIAN_POINT('',(15.,-20.5,-10.75));
#23266=CARTESIAN_POINT('Origin',(13.5,-20.5,18.));
#23267=CARTESIAN_POINT('Origin',(70.,-22.,-25.));
#23268=CARTESIAN_POINT('',(13.5,-22.,-25.));
#23269=CARTESIAN_POINT('Origin',(13.5,-22.,-23.5));
#23270=CARTESIAN_POINT('',(15.,-22.,-23.5));
#23271=CARTESIAN_POINT('Origin',(13.5,20.5,-10.75));
#23272=CARTESIAN_POINT('',(13.5,22.,18.));
#23273=CARTESIAN_POINT('',(13.5,22.,-10.75));
#23274=CARTESIAN_POINT('',(15.,20.5,18.));
#23275=CARTESIAN_POINT('Origin',(13.5,20.5,18.));
#23276=CARTESIAN_POINT('',(15.,20.5,-10.75));
#23277=CARTESIAN_POINT('Origin',(24.,-20.5,40.5));
#23278=CARTESIAN_POINT('Origin',(82.5,-20.5,15.25));
#23279=CARTESIAN_POINT('',(84.,-20.5,17.5712833908056));
#23280=CARTESIAN_POINT('Ctrl Pts',(84.,-20.5,17.5712833908056));
#23281=CARTESIAN_POINT('Ctrl Pts',(84.,-20.7022477383282,17.3353257465337));
#23282=CARTESIAN_POINT('Ctrl Pts',(83.9575260447373,-20.9170846786411,17.0756837501162));
#23283=CARTESIAN_POINT('Ctrl Pts',(83.7765132729403,-21.3178359703858,16.572666547787));
#23284=CARTESIAN_POINT('Ctrl Pts',(83.6391148171733,-21.5040391092436,16.3291117577357));
#23285=CARTESIAN_POINT('Ctrl Pts',(83.3468785813891,-21.7463710185311,16.0037159774975));
#23286=CARTESIAN_POINT('Ctrl Pts',(83.2051881089356,-21.8355590404292,15.88144036437));
#23287=CARTESIAN_POINT('Ctrl Pts',(82.9588244922017,-21.9308152339295,15.7493583883479));
#23288=CARTESIAN_POINT('Ctrl Pts',(82.8710686191993,-21.9563375109926,15.7136914161295));
#23289=CARTESIAN_POINT('Ctrl Pts',(82.6889643978921,-21.9909261474626,15.665250854624));
#23290=CARTESIAN_POINT('Ctrl Pts',(82.5946178513886,-22.,15.6524758424985));
#23291=CARTESIAN_POINT('Ctrl Pts',(82.5,-22.,15.6524758424985));
#23292=CARTESIAN_POINT('',(84.,-20.5,15.25));
#23293=CARTESIAN_POINT('Origin',(84.,-22.,22.));
#23294=CARTESIAN_POINT('Origin',(84.,0.,0.));
#23295=CARTESIAN_POINT('Origin',(70.,-22.,0.));
#23296=CARTESIAN_POINT('Origin',(70.,0.,0.));
#23297=CARTESIAN_POINT('Origin',(61.5,-20.5,14.75));
#23298=CARTESIAN_POINT('',(61.5,-22.,-15.6524758424985));
#23299=CARTESIAN_POINT('',(61.5,-22.,14.75));
#23300=CARTESIAN_POINT('Ctrl Pts',(60.,-20.5,-15.1657508881031));
#23301=CARTESIAN_POINT('Ctrl Pts',(60.,-20.5020625379506,-15.1664308867282));
#23302=CARTESIAN_POINT('Ctrl Pts',(60.0000042540628,-20.5041250881598,-15.1671108436611));
#23303=CARTESIAN_POINT('Ctrl Pts',(60.000459532602,-20.6144922519149,-15.2034929264267));
#23304=CARTESIAN_POINT('Ctrl Pts',(60.0126356314555,-20.7225920605635,-15.2390001138621));
#23305=CARTESIAN_POINT('Ctrl Pts',(60.0601510385376,-20.9342353436599,-15.3082836950208));
#23306=CARTESIAN_POINT('Ctrl Pts',(60.0953241933879,-21.0373769241961,-15.3419294911594));
#23307=CARTESIAN_POINT('Ctrl Pts',(60.2231667795538,-21.310385626032,-15.4307183360865));
#23308=CARTESIAN_POINT('Ctrl Pts',(60.3382746523712,-21.4688874023992,-15.4819477371951));
#23309=CARTESIAN_POINT('Ctrl Pts',(60.6191603261817,-21.7283867354349,-15.5655237678324));
#23310=CARTESIAN_POINT('Ctrl Pts',(60.7797547588616,-21.8293573646189,-15.5978863073161));
#23311=CARTESIAN_POINT('Ctrl Pts',(61.129199035605,-21.9652152818212,-15.6413750983628));
#23312=CARTESIAN_POINT('Ctrl Pts',(61.3134705059138,-22.,-15.6524758424985));
#23313=CARTESIAN_POINT('Ctrl Pts',(61.5,-22.,-15.6524758424985));
#23314=CARTESIAN_POINT('Origin',(61.5,-22.,-23.5));
#23315=CARTESIAN_POINT('Ctrl Pts',(61.5,-10.1980390271856,-25.));
#23316=CARTESIAN_POINT('Ctrl Pts',(61.3081176819558,-10.1980390271856,-25.));
#23317=CARTESIAN_POINT('Ctrl Pts',(61.1182675528468,-10.1908261217545,-24.9631850847576));
#23318=CARTESIAN_POINT('Ctrl Pts',(60.7614154879323,-10.1626433260876,-24.8197797335775));
#23319=CARTESIAN_POINT('Ctrl Pts',(60.5983542509472,-10.1418364073688,-24.7140382945063));
#23320=CARTESIAN_POINT('Ctrl Pts',(60.3189691603886,-10.0886902105648,-24.4452375771159));
#23321=CARTESIAN_POINT('Ctrl Pts',(60.2063475813541,-10.0566512843893,-24.283743850747));
#23322=CARTESIAN_POINT('Ctrl Pts',(60.0861774650203,-10.0023374403617,-24.0115999983853));
#23323=CARTESIAN_POINT('Ctrl Pts',(60.054419379683,-9.98267886135603,-23.9133673884351));
#23324=CARTESIAN_POINT('Ctrl Pts',(60.0114978161663,-9.94226557571909,-23.7120589639788));
#23325=CARTESIAN_POINT('Ctrl Pts',(60.0004641001801,-9.92160226317557,-23.6094398880042));
#23326=CARTESIAN_POINT('Ctrl Pts',(60.0000047777623,-9.90037810810563,-23.504371622114));
#23327=CARTESIAN_POINT('Ctrl Pts',(60.,-9.8999365367755,-23.5021858092929));
#23328=CARTESIAN_POINT('Ctrl Pts',(60.,-9.89949493661168,-23.5));
#23329=CARTESIAN_POINT('Origin',(42.,-22.,8.5));
#23330=CARTESIAN_POINT('',(75.5,-22.,-15.6524758424985));
#23331=CARTESIAN_POINT('Origin',(61.5,20.5,-23.5));
#23332=CARTESIAN_POINT('',(61.5,20.5,-25.));
#23333=CARTESIAN_POINT('',(61.5,22.,-23.5));
#23334=CARTESIAN_POINT('Origin',(61.5,20.5,-23.5));
#23335=CARTESIAN_POINT('Origin',(61.5,20.5,-23.5));
#23336=CARTESIAN_POINT('Origin',(61.5,20.5,-23.5));
#23337=CARTESIAN_POINT('Origin',(61.5,-22.,-23.5));
#23338=CARTESIAN_POINT('',(61.5,10.1980390271856,-25.));
#23339=CARTESIAN_POINT('Ctrl Pts',(60.,9.89949493661168,-23.5));
#23340=CARTESIAN_POINT('Ctrl Pts',(60.,9.89993832731204,-23.5021946719966));
#23341=CARTESIAN_POINT('Ctrl Pts',(60.0000048165852,9.90038168894123,-23.5043893475508));
#23342=CARTESIAN_POINT('Ctrl Pts',(60.0004660319782,9.92160723858752,-23.6094645739685));
#23343=CARTESIAN_POINT('Ctrl Pts',(60.0115011689912,9.94227012456818,-23.7120815813529));
#23344=CARTESIAN_POINT('Ctrl Pts',(60.0544249797747,9.98268274401981,-23.9133867704278));
#23345=CARTESIAN_POINT('Ctrl Pts',(60.0861841059616,10.0023410769715,-24.0116181880972));
#23346=CARTESIAN_POINT('Ctrl Pts',(60.206355943955,10.0566538664141,-24.2837568481804));
#23347=CARTESIAN_POINT('Ctrl Pts',(60.3189770792875,10.0886920356348,-24.4452467916769));
#23348=CARTESIAN_POINT('Ctrl Pts',(60.5983596493521,10.1418371216814,-24.7140419232243));
#23349=CARTESIAN_POINT('Ctrl Pts',(60.7614191687488,10.1626436608923,-24.819781436362));
#23350=CARTESIAN_POINT('Ctrl Pts',(61.1182686232222,10.1908261625926,-24.9631852933862));
#23351=CARTESIAN_POINT('Ctrl Pts',(61.3081182257788,10.1980390271856,-25.));
#23352=CARTESIAN_POINT('Ctrl Pts',(61.5,10.1980390271856,-25.));
#23353=CARTESIAN_POINT('',(61.5,-22.,-25.));
#23354=CARTESIAN_POINT('Origin',(61.5,20.5,14.75));
#23355=CARTESIAN_POINT('',(61.5,22.,-15.6524758424985));
#23356=CARTESIAN_POINT('Ctrl Pts',(61.5,22.,-15.6524758424985));
#23357=CARTESIAN_POINT('Ctrl Pts',(61.3134858239941,22.,-15.6524758424985));
#23358=CARTESIAN_POINT('Ctrl Pts',(61.1292291179574,21.9652209916066,-15.6413769188859));
#23359=CARTESIAN_POINT('Ctrl Pts',(60.7798600570244,21.8294044226054,-15.5979013781792));
#23360=CARTESIAN_POINT('Ctrl Pts',(60.619315251053,21.7284875323288,-15.5655560876705));
#23361=CARTESIAN_POINT('Ctrl Pts',(60.3385094668615,21.4691487038552,-15.482032043976));
#23362=CARTESIAN_POINT('Ctrl Pts',(60.2234187980134,21.3107595052867,-15.4308393408124));
#23363=CARTESIAN_POINT('Ctrl Pts',(60.0954774955618,21.0377971691356,-15.3420664979276));
#23364=CARTESIAN_POINT('Ctrl Pts',(60.0602457537108,20.9345730436471,-15.3083940597981));
#23365=CARTESIAN_POINT('Ctrl Pts',(60.0126604270431,20.7227867271798,-15.239064024796));
#23366=CARTESIAN_POINT('Ctrl Pts',(60.0004657094814,20.6146288648013,-15.2035378999918));
#23367=CARTESIAN_POINT('Ctrl Pts',(60.0000043615329,20.5041768692451,-15.1671279142233));
#23368=CARTESIAN_POINT('Ctrl Pts',(60.,20.502088428345,-15.1664394225385));
#23369=CARTESIAN_POINT('Ctrl Pts',(60.,20.5,-15.1657508881031));
#23370=CARTESIAN_POINT('',(61.5,22.,14.75));
#23371=CARTESIAN_POINT('Origin',(68.5,20.5,-23.5));
#23372=CARTESIAN_POINT('',(68.5,20.5,-25.));
#23373=CARTESIAN_POINT('',(68.5,22.,-23.5));
#23374=CARTESIAN_POINT('Origin',(68.5,20.5,-23.5));
#23375=CARTESIAN_POINT('',(70.,20.5,-23.5));
#23376=CARTESIAN_POINT('Origin',(68.5,20.5,-23.5));
#23377=CARTESIAN_POINT('Origin',(68.5,20.5,-23.5));
#23378=CARTESIAN_POINT('Origin',(56.,20.5,-23.5));
#23379=CARTESIAN_POINT('',(56.,20.5,-25.));
#23380=CARTESIAN_POINT('',(56.,22.,-23.5));
#23381=CARTESIAN_POINT('Origin',(70.,-22.,-25.));
#23382=CARTESIAN_POINT('',(68.5,10.1980390271856,-25.));
#23383=CARTESIAN_POINT('',(68.5,-22.,-25.));
#23384=CARTESIAN_POINT('',(75.5,10.1980390271856,-25.));
#23385=CARTESIAN_POINT('Origin',(68.5,-22.,-23.5));
#23386=CARTESIAN_POINT('',(70.,13.2947358003083,-23.5));
#23387=CARTESIAN_POINT('',(70.,-22.,-23.5));
#23388=CARTESIAN_POINT('Ctrl Pts',(68.5,10.1980390271856,-25.));
#23389=CARTESIAN_POINT('Ctrl Pts',(68.5690622745619,10.1980390271856,-25.));
#23390=CARTESIAN_POINT('Ctrl Pts',(68.64269539724,10.2107026186997,-24.9948442089972));
#23391=CARTESIAN_POINT('Ctrl Pts',(68.7815873963742,10.2591413018302,-24.97500159694));
#23392=CARTESIAN_POINT('Ctrl Pts',(68.8470061948633,10.2945164376804,-24.9604604345961));
#23393=CARTESIAN_POINT('Ctrl Pts',(69.099996626182,10.4648018594106,-24.889928820497));
#23394=CARTESIAN_POINT('Ctrl Pts',(69.2682778073745,10.6853817343331,-24.7965377420129));
#23395=CARTESIAN_POINT('Ctrl Pts',(69.8122976763679,11.5896482415098,-24.3983540225569));
#23396=CARTESIAN_POINT('Ctrl Pts',(70.,12.5253526611459,-23.9352657686969));
#23397=CARTESIAN_POINT('Ctrl Pts',(70.,13.2947358003083,-23.5));
#23398=CARTESIAN_POINT('Origin',(68.5,20.5,4.25));
#23399=CARTESIAN_POINT('',(68.5,22.,-15.6524758424985));
#23400=CARTESIAN_POINT('',(68.5,22.,4.25));
#23401=CARTESIAN_POINT('',(70.,20.5,-17.5712833908056));
#23402=CARTESIAN_POINT('Ctrl Pts',(70.,20.5,-17.5712833908056));
#23403=CARTESIAN_POINT('Ctrl Pts',(70.,20.7022477383282,-17.3353257465337));
#23404=CARTESIAN_POINT('Ctrl Pts',(69.9575260447372,20.9170846786411,-17.0756837501162));
#23405=CARTESIAN_POINT('Ctrl Pts',(69.7765132729404,21.3178359703858,-16.572666547787));
#23406=CARTESIAN_POINT('Ctrl Pts',(69.6391148171733,21.5040391092436,-16.3291117577357));
#23407=CARTESIAN_POINT('Ctrl Pts',(69.3468785813891,21.7463710185311,-16.0037159774975));
#23408=CARTESIAN_POINT('Ctrl Pts',(69.2051881089356,21.8355590404292,-15.88144036437));
#23409=CARTESIAN_POINT('Ctrl Pts',(68.9588244922017,21.9308152339295,-15.7493583883479));
#23410=CARTESIAN_POINT('Ctrl Pts',(68.8710686191993,21.9563375109926,-15.7136914161295));
#23411=CARTESIAN_POINT('Ctrl Pts',(68.6889643978921,21.9909261474626,-15.665250854624));
#23412=CARTESIAN_POINT('Ctrl Pts',(68.5946178513885,22.,-15.6524758424985));
#23413=CARTESIAN_POINT('Ctrl Pts',(68.5,22.,-15.6524758424985));
#23414=CARTESIAN_POINT('',(70.,20.5,4.25));
#23415=CARTESIAN_POINT('Origin',(70.,-22.,0.));
#23416=CARTESIAN_POINT('Origin',(70.,0.,0.));
#23417=CARTESIAN_POINT('Origin',(90.5,0.,0.));
#23418=CARTESIAN_POINT('',(92.,-3.10799188078457E-15,25.3786796564404));
#23419=CARTESIAN_POINT('Origin',(92.,0.,0.));
#23420=CARTESIAN_POINT('',(91.5606601717798,-3.2378852892199E-15,26.4393398282202));
#23421=CARTESIAN_POINT('Origin',(90.5,-3.10799188078457E-15,25.3786796564404));
#23422=CARTESIAN_POINT('',(91.5606601717798,-26.4393398282202,-3.2378852892199E-15));
#23423=CARTESIAN_POINT('Origin',(91.5606601717798,0.,-4.04735661152487E-15));
#23424=CARTESIAN_POINT('Origin',(91.5606601717798,0.,-4.04735661152487E-15));
#23425=CARTESIAN_POINT('Origin',(91.5,0.,0.));
#23426=CARTESIAN_POINT('',(91.4393398282202,-26.5606601717798,-3.25274274626107E-15));
#23427=CARTESIAN_POINT('',(91.5,-26.5,-3.24531401774049E-15));
#23428=CARTESIAN_POINT('',(91.4393398282202,-3.25274274626107E-15,26.5606601717798));
#23429=CARTESIAN_POINT('Origin',(91.4393398282202,0.,-4.06592843282634E-15));
#23430=CARTESIAN_POINT('Origin',(91.4393398282202,0.,-4.06592843282634E-15));
#23431=CARTESIAN_POINT('Origin',(92.,0.,0.));
#23432=CARTESIAN_POINT('',(92.,-21.905,2.68258881353228E-15));
#23433=CARTESIAN_POINT('Origin',(92.,0.,0.));
#23434=CARTESIAN_POINT('Origin',(90.3786796564403,0.,0.));
#23435=CARTESIAN_POINT('',(90.3786796564403,-3.30654635769785E-15,27.));
#23436=CARTESIAN_POINT('Origin',(90.3786796564403,-3.12284933782575E-15,
25.5));
#23437=CARTESIAN_POINT('',(90.3786796564403,-27.,-3.30654635769785E-15));
#23438=CARTESIAN_POINT('Origin',(90.3786796564403,0.,0.));
#23439=CARTESIAN_POINT('Origin',(90.3786796564403,0.,0.));
#23440=CARTESIAN_POINT('Origin',(75.5,0.,0.));
#23441=CARTESIAN_POINT('',(61.5,-27.,-3.30654635769785E-15));
#23442=CARTESIAN_POINT('',(75.5,-27.,-3.30654635769785E-15));
#23443=CARTESIAN_POINT('Origin',(61.5,0.,0.));
#23444=CARTESIAN_POINT('Origin',(61.5,0.,0.));
#23445=CARTESIAN_POINT('',(75.5,22.,-15.6524758424985));
#23446=CARTESIAN_POINT('',(61.5,22.,15.6524758424985));
#23447=CARTESIAN_POINT('Origin',(61.5,0.,0.));
#23448=CARTESIAN_POINT('',(75.5,22.,15.6524758424985));
#23449=CARTESIAN_POINT('Origin',(84.,0.,0.));
#23450=CARTESIAN_POINT('Origin',(61.5,0.,0.));
#23451=CARTESIAN_POINT('Origin',(61.5,0.,0.));
#23452=CARTESIAN_POINT('Origin',(28.5,20.5,22.5));
#23453=CARTESIAN_POINT('',(57.,22.,22.5));
#23454=CARTESIAN_POINT('',(57.,20.5,21.));
#23455=CARTESIAN_POINT('Origin',(57.,20.5,22.5));
#23456=CARTESIAN_POINT('',(18.,20.5,21.));
#23457=CARTESIAN_POINT('',(28.5,20.5,21.));
#23458=CARTESIAN_POINT('',(18.,22.,22.5));
#23459=CARTESIAN_POINT('Origin',(18.,20.5,22.5));
#23460=CARTESIAN_POINT('',(28.5,22.,22.5));
#23461=CARTESIAN_POINT('Origin',(18.,20.5,18.));
#23462=CARTESIAN_POINT('Origin',(18.,22.,18.));
#23463=CARTESIAN_POINT('Origin',(18.,20.5,18.));
#23464=CARTESIAN_POINT('Origin',(28.5,-20.5,22.5));
#23465=CARTESIAN_POINT('',(18.,-20.5,21.));
#23466=CARTESIAN_POINT('Origin',(18.,-20.5,22.5));
#23467=CARTESIAN_POINT('',(57.,-20.5,21.));
#23468=CARTESIAN_POINT('',(28.5,-20.5,21.));
#23469=CARTESIAN_POINT('Origin',(57.,-20.5,22.5));
#23470=CARTESIAN_POINT('Origin',(57.,-20.5,18.));
#23471=CARTESIAN_POINT('Origin',(61.5,-20.5,18.));
#23472=CARTESIAN_POINT('Origin',(57.,-20.5,18.));
#23473=CARTESIAN_POINT('Origin',(61.5,-20.5,14.75));
#23474=CARTESIAN_POINT('Ctrl Pts',(60.,-20.5,15.1657508881031));
#23475=CARTESIAN_POINT('Ctrl Pts',(60.,-20.5018310939024,15.1663545818852));
#23476=CARTESIAN_POINT('Ctrl Pts',(60.0000033529049,-20.5036621975828,15.1669582428458));
#23477=CARTESIAN_POINT('Ctrl Pts',(60.0004057833521,-20.6135490452472,15.2031825380108));
#23478=CARTESIAN_POINT('Ctrl Pts',(60.0124770444123,-20.7214063029217,15.2386108915177));
#23479=CARTESIAN_POINT('Ctrl Pts',(60.0596389516904,-20.9324251256081,15.3076921352536));
#23480=CARTESIAN_POINT('Ctrl Pts',(60.0945262837795,-21.0351965386236,15.3412186660997));
#23481=CARTESIAN_POINT('Ctrl Pts',(60.2218896363614,-21.3084881625076,15.430104219162));
#23482=CARTESIAN_POINT('Ctrl Pts',(60.3370862252174,-21.4675640567846,15.4815207668313));
#23483=CARTESIAN_POINT('Ctrl Pts',(60.6183791948953,-21.7278782657557,15.5653607304813));
#23484=CARTESIAN_POINT('Ctrl Pts',(60.7792244100121,-21.8291204213603,15.5978104235522));
#23485=CARTESIAN_POINT('Ctrl Pts',(61.1290483151644,-21.9651866670112,15.6413659747481));
#23486=CARTESIAN_POINT('Ctrl Pts',(61.3133937576427,-22.,15.6524758424985));
#23487=CARTESIAN_POINT('Ctrl Pts',(61.5,-22.,15.6524758424985));
#23488=CARTESIAN_POINT('Origin',(18.,-20.5,18.));
#23489=CARTESIAN_POINT('Origin',(18.,-20.5,18.));
#23490=CARTESIAN_POINT('Origin',(61.5,0.,0.));
#23491=CARTESIAN_POINT('Origin',(57.,20.5,18.));
#23492=CARTESIAN_POINT('',(61.5,22.,18.));
#23493=CARTESIAN_POINT('Origin',(61.5,20.5,18.));
#23494=CARTESIAN_POINT('Origin',(57.,20.5,18.));
#23495=CARTESIAN_POINT('Origin',(57.,22.,18.));
#23496=CARTESIAN_POINT('Origin',(61.5,20.5,14.75));
#23497=CARTESIAN_POINT('',(61.5,22.,14.75));
#23498=CARTESIAN_POINT('Ctrl Pts',(61.5,22.,15.6524758424985));
#23499=CARTESIAN_POINT('Ctrl Pts',(61.3133937576427,22.,15.6524758424985));
#23500=CARTESIAN_POINT('Ctrl Pts',(61.1290483151644,21.9651866670112,15.6413659747481));
#23501=CARTESIAN_POINT('Ctrl Pts',(60.7792244100121,21.8291204213603,15.5978104235522));
#23502=CARTESIAN_POINT('Ctrl Pts',(60.6183791948954,21.7278782657557,15.5653607304813));
#23503=CARTESIAN_POINT('Ctrl Pts',(60.3370862252174,21.4675640567846,15.4815207668312));
#23504=CARTESIAN_POINT('Ctrl Pts',(60.2218896363614,21.3084881625076,15.430104219162));
#23505=CARTESIAN_POINT('Ctrl Pts',(60.0945262837793,21.0351965386233,15.3412186660996));
#23506=CARTESIAN_POINT('Ctrl Pts',(60.0596389516902,20.9324251256073,15.3076921352533));
#23507=CARTESIAN_POINT('Ctrl Pts',(60.0124770444122,20.7214063029204,15.2386108915173));
#23508=CARTESIAN_POINT('Ctrl Pts',(60.0004057833519,20.613549045247,15.2031825380104));
#23509=CARTESIAN_POINT('Ctrl Pts',(60.0000033529049,20.5036621975811,15.1669582428453));
#23510=CARTESIAN_POINT('Ctrl Pts',(60.,20.5018310939017,15.166354581885));
#23511=CARTESIAN_POINT('Ctrl Pts',(60.,20.5,15.1657508881031));
#23512=CARTESIAN_POINT('Origin',(61.5,0.,0.));
#23513=CARTESIAN_POINT('Origin',(15.,-22.,-30.));
#23514=CARTESIAN_POINT('',(15.,-22.,18.));
#23515=CARTESIAN_POINT('',(15.,-3.73517273739943E-16,3.05));
#23516=CARTESIAN_POINT('Origin',(15.,0.,0.));
#23517=CARTESIAN_POINT('Origin',(18.,-22.,18.));
#23518=CARTESIAN_POINT('',(18.,-22.,21.));
#23519=CARTESIAN_POINT('Origin',(15.,-22.,21.));
#23520=CARTESIAN_POINT('',(57.,-22.,21.));
#23521=CARTESIAN_POINT('Origin',(57.,-22.,18.));
#23522=CARTESIAN_POINT('Ctrl Pts',(32.5358115136623,-2.58526623249054,42.));
#23523=CARTESIAN_POINT('Ctrl Pts',(32.5358115136623,-2.58526623249054,41.7));
#23524=CARTESIAN_POINT('Ctrl Pts',(31.8298088014126,-2.58526623249054,42.));
#23525=CARTESIAN_POINT('Ctrl Pts',(31.8298088014126,-2.58526623249054,41.7));
#23526=CARTESIAN_POINT('Ctrl Pts',(31.2738743424416,-2.24420189857483,42.));
#23527=CARTESIAN_POINT('Ctrl Pts',(31.2738743424416,-2.24420189857483,41.7));
#23528=CARTESIAN_POINT('',(32.5358115136623,-2.58526623249054,41.7));
#23529=CARTESIAN_POINT('',(32.5358115136623,-2.58526623249054,42.));
#23530=CARTESIAN_POINT('',(31.2738743424416,-2.24420189857483,41.7));
#23531=CARTESIAN_POINT('Ctrl Pts',(32.5358115136623,-2.58526623249054,41.7));
#23532=CARTESIAN_POINT('Ctrl Pts',(31.8298088014126,-2.58526623249054,41.7));
#23533=CARTESIAN_POINT('Ctrl Pts',(31.2738743424416,-2.24420189857483,41.7));
#23534=CARTESIAN_POINT('',(31.2738743424416,-2.24420189857483,42.));
#23535=CARTESIAN_POINT('Ctrl Pts',(33.7499998509884,-2.27660298347473,42.));
#23536=CARTESIAN_POINT('Ctrl Pts',(33.7499998509884,-2.27660298347473,41.7));
#23537=CARTESIAN_POINT('Ctrl Pts',(33.1872440874577,-2.58526623249054,42.));
#23538=CARTESIAN_POINT('Ctrl Pts',(33.1872440874577,-2.58526623249054,41.7));
#23539=CARTESIAN_POINT('Ctrl Pts',(32.5358115136623,-2.58526623249054,42.));
#23540=CARTESIAN_POINT('Ctrl Pts',(32.5358115136623,-2.58526623249054,41.7));
#23541=CARTESIAN_POINT('',(33.7499998509884,-2.27660298347473,41.7));
#23542=CARTESIAN_POINT('',(33.7499998509884,-2.27660298347473,42.));
#23543=CARTESIAN_POINT('Ctrl Pts',(33.7499998509884,-2.27660298347473,41.7));
#23544=CARTESIAN_POINT('Ctrl Pts',(33.1872440874577,-2.58526623249054,41.7));
#23545=CARTESIAN_POINT('Ctrl Pts',(32.5358115136623,-2.58526623249054,41.7));
#23546=CARTESIAN_POINT('Ctrl Pts',(34.6197132766247,-1.36766731739044,42.));
#23547=CARTESIAN_POINT('Ctrl Pts',(34.6197132766247,-1.36766731739044,41.7));
#23548=CARTESIAN_POINT('Ctrl Pts',(34.3127556145191,-1.96793973445892,42.));
#23549=CARTESIAN_POINT('Ctrl Pts',(34.3127556145191,-1.96793973445892,41.7));
#23550=CARTESIAN_POINT('Ctrl Pts',(33.7499998509884,-2.27660298347473,42.));
#23551=CARTESIAN_POINT('Ctrl Pts',(33.7499998509884,-2.27660298347473,41.7));
#23552=CARTESIAN_POINT('',(34.6197132766247,-1.36766731739044,41.7));
#23553=CARTESIAN_POINT('',(34.6197132766247,-1.36766731739044,42.));
#23554=CARTESIAN_POINT('Ctrl Pts',(34.6197132766247,-1.36766731739044,41.7));
#23555=CARTESIAN_POINT('Ctrl Pts',(34.3127556145191,-1.96793973445892,41.7));
#23556=CARTESIAN_POINT('Ctrl Pts',(33.7499998509884,-2.27660298347473,41.7));
#23557=CARTESIAN_POINT('Ctrl Pts',(34.9266712367535,-0.00682175159454346,
42.));
#23558=CARTESIAN_POINT('Ctrl Pts',(34.9266712367535,-0.00682175159454346,
41.7));
#23559=CARTESIAN_POINT('Ctrl Pts',(34.9266712367535,-0.767394304275513,
42.));
#23560=CARTESIAN_POINT('Ctrl Pts',(34.9266712367535,-0.767394304275513,
41.7));
#23561=CARTESIAN_POINT('Ctrl Pts',(34.6197132766247,-1.36766731739044,42.));
#23562=CARTESIAN_POINT('Ctrl Pts',(34.6197132766247,-1.36766731739044,41.7));
#23563=CARTESIAN_POINT('',(34.9266712367535,-0.00682175159454346,41.7));
#23564=CARTESIAN_POINT('',(34.9266712367535,-0.00682175159454346,42.));
#23565=CARTESIAN_POINT('Ctrl Pts',(34.9266712367535,-0.00682175159454346,
41.7));
#23566=CARTESIAN_POINT('Ctrl Pts',(34.9266712367535,-0.767394304275513,
41.7));
#23567=CARTESIAN_POINT('Ctrl Pts',(34.6197132766247,-1.36766731739044,41.7));
#23568=CARTESIAN_POINT('Ctrl Pts',(34.6350611746311,1.33526593446732,42.));
#23569=CARTESIAN_POINT('Ctrl Pts',(34.6350611746311,1.33526593446732,41.7));
#23570=CARTESIAN_POINT('Ctrl Pts',(34.9266712367535,0.74351966381073,42.));
#23571=CARTESIAN_POINT('Ctrl Pts',(34.9266712367535,0.74351966381073,41.7));
#23572=CARTESIAN_POINT('Ctrl Pts',(34.9266712367535,-0.00682175159454346,
42.));
#23573=CARTESIAN_POINT('Ctrl Pts',(34.9266712367535,-0.00682175159454346,
41.7));
#23574=CARTESIAN_POINT('',(34.6350611746311,1.33526593446732,41.7));
#23575=CARTESIAN_POINT('',(34.6350611746311,1.33526593446732,42.));
#23576=CARTESIAN_POINT('Ctrl Pts',(34.6350611746311,1.33526593446732,41.7));
#23577=CARTESIAN_POINT('Ctrl Pts',(34.9266712367535,0.74351966381073,41.7));
#23578=CARTESIAN_POINT('Ctrl Pts',(34.9266712367535,-0.00682175159454346,
41.7));
#23579=CARTESIAN_POINT('Ctrl Pts',(33.7875168025494,2.25784420967102,42.));
#23580=CARTESIAN_POINT('Ctrl Pts',(33.7875168025494,2.25784420967102,41.7));
#23581=CARTESIAN_POINT('Ctrl Pts',(34.343451410532,1.92701190710068,42.));
#23582=CARTESIAN_POINT('Ctrl Pts',(34.343451410532,1.92701190710068,41.7));
#23583=CARTESIAN_POINT('Ctrl Pts',(34.6350611746311,1.33526593446732,42.));
#23584=CARTESIAN_POINT('Ctrl Pts',(34.6350611746311,1.33526593446732,41.7));
#23585=CARTESIAN_POINT('',(33.7875168025494,2.25784420967102,41.7));
#23586=CARTESIAN_POINT('',(33.7875168025494,2.25784420967102,42.));
#23587=CARTESIAN_POINT('Ctrl Pts',(33.7875168025494,2.25784420967102,41.7));
#23588=CARTESIAN_POINT('Ctrl Pts',(34.343451410532,1.92701190710068,41.7));
#23589=CARTESIAN_POINT('Ctrl Pts',(34.6350611746311,1.33526593446732,41.7));
#23590=CARTESIAN_POINT('Ctrl Pts',(32.5392223894596,2.58867621421814,42.));
#23591=CARTESIAN_POINT('Ctrl Pts',(32.5392223894596,2.58867621421814,41.7));
#23592=CARTESIAN_POINT('Ctrl Pts',(33.23158249259,2.58867621421814,42.));
#23593=CARTESIAN_POINT('Ctrl Pts',(33.23158249259,2.58867621421814,41.7));
#23594=CARTESIAN_POINT('Ctrl Pts',(33.7875168025494,2.25784420967102,42.));
#23595=CARTESIAN_POINT('Ctrl Pts',(33.7875168025494,2.25784420967102,41.7));
#23596=CARTESIAN_POINT('',(32.5392223894596,2.58867621421814,41.7));
#23597=CARTESIAN_POINT('',(32.5392223894596,2.58867621421814,42.));
#23598=CARTESIAN_POINT('Ctrl Pts',(32.5392223894596,2.58867621421814,41.7));
#23599=CARTESIAN_POINT('Ctrl Pts',(33.23158249259,2.58867621421814,41.7));
#23600=CARTESIAN_POINT('Ctrl Pts',(33.7875168025494,2.25784420967102,41.7));
#23601=CARTESIAN_POINT('Ctrl Pts',(30.8134378492832,1.88437908887863,42.));
#23602=CARTESIAN_POINT('Ctrl Pts',(30.8134378492832,1.88437908887863,41.7));
#23603=CARTESIAN_POINT('Ctrl Pts',(31.4819234609604,2.58867621421814,42.));
#23604=CARTESIAN_POINT('Ctrl Pts',(31.4819234609604,2.58867621421814,41.7));
#23605=CARTESIAN_POINT('Ctrl Pts',(32.5392223894596,2.58867621421814,42.));
#23606=CARTESIAN_POINT('Ctrl Pts',(32.5392223894596,2.58867621421814,41.7));
#23607=CARTESIAN_POINT('',(30.8134378492832,1.88437908887863,41.7));
#23608=CARTESIAN_POINT('',(30.8134378492832,1.88437908887863,42.));
#23609=CARTESIAN_POINT('Ctrl Pts',(30.8134378492832,1.88437908887863,41.7));
#23610=CARTESIAN_POINT('Ctrl Pts',(31.4819234609604,2.58867621421814,41.7));
#23611=CARTESIAN_POINT('Ctrl Pts',(32.5392223894596,2.58867621421814,41.7));
#23612=CARTESIAN_POINT('Ctrl Pts',(30.1449521258473,-0.0648021697998047,
42.));
#23613=CARTESIAN_POINT('Ctrl Pts',(30.1449521258473,-0.0648021697998047,
41.7));
#23614=CARTESIAN_POINT('Ctrl Pts',(30.1449521258473,1.1800816655159,42.));
#23615=CARTESIAN_POINT('Ctrl Pts',(30.1449521258473,1.1800816655159,41.7));
#23616=CARTESIAN_POINT('Ctrl Pts',(30.8134378492832,1.88437908887863,42.));
#23617=CARTESIAN_POINT('Ctrl Pts',(30.8134378492832,1.88437908887863,41.7));
#23618=CARTESIAN_POINT('',(30.1449521258473,-0.0648021697998047,41.7));
#23619=CARTESIAN_POINT('',(30.1449521258473,-0.0648021697998047,42.));
#23620=CARTESIAN_POINT('Ctrl Pts',(30.1449521258473,-0.0648021697998047,
41.7));
#23621=CARTESIAN_POINT('Ctrl Pts',(30.1449521258473,1.1800816655159,41.7));
#23622=CARTESIAN_POINT('Ctrl Pts',(30.8134378492832,1.88437908887863,41.7));
#23623=CARTESIAN_POINT('Ctrl Pts',(30.4314459860325,-1.31309688091278,42.));
#23624=CARTESIAN_POINT('Ctrl Pts',(30.4314459860325,-1.31309688091278,41.7));
#23625=CARTESIAN_POINT('Ctrl Pts',(30.1449521258473,-0.723056197166443,
42.));
#23626=CARTESIAN_POINT('Ctrl Pts',(30.1449521258473,-0.723056197166443,
41.7));
#23627=CARTESIAN_POINT('Ctrl Pts',(30.1449521258473,-0.0648021697998047,
42.));
#23628=CARTESIAN_POINT('Ctrl Pts',(30.1449521258473,-0.0648021697998047,
41.7));
#23629=CARTESIAN_POINT('',(30.4314459860325,-1.31309688091278,41.7));
#23630=CARTESIAN_POINT('',(30.4314459860325,-1.31309688091278,42.));
#23631=CARTESIAN_POINT('Ctrl Pts',(30.4314459860325,-1.31309688091278,41.7));
#23632=CARTESIAN_POINT('Ctrl Pts',(30.1449521258473,-0.723056197166443,
41.7));
#23633=CARTESIAN_POINT('Ctrl Pts',(30.1449521258473,-0.0648021697998047,
41.7));
#23634=CARTESIAN_POINT('Ctrl Pts',(31.2738743424416,-2.24420189857483,42.));
#23635=CARTESIAN_POINT('Ctrl Pts',(31.2738743424416,-2.24420189857483,41.7));
#23636=CARTESIAN_POINT('Ctrl Pts',(30.7179398834705,-1.90313756465912,42.));
#23637=CARTESIAN_POINT('Ctrl Pts',(30.7179398834705,-1.90313756465912,41.7));
#23638=CARTESIAN_POINT('Ctrl Pts',(30.4314459860325,-1.31309688091278,42.));
#23639=CARTESIAN_POINT('Ctrl Pts',(30.4314459860325,-1.31309688091278,41.7));
#23640=CARTESIAN_POINT('Ctrl Pts',(31.2738743424416,-2.24420189857483,41.7));
#23641=CARTESIAN_POINT('Ctrl Pts',(30.7179398834705,-1.90313756465912,41.7));
#23642=CARTESIAN_POINT('Ctrl Pts',(30.4314459860325,-1.31309688091278,41.7));
#23643=CARTESIAN_POINT('Origin',(32.5358116813004,0.00170499086380005,41.7));
#23644=CARTESIAN_POINT('Origin',(29.667462259531,1.90995901823044,42.));
#23645=CARTESIAN_POINT('',(29.667462259531,1.90995901823044,41.7));
#23646=CARTESIAN_POINT('',(29.667462259531,1.90995901823044,42.));
#23647=CARTESIAN_POINT('',(28.0133013427258,1.90995901823044,41.7));
#23648=CARTESIAN_POINT('',(29.667462259531,1.90995901823044,41.7));
#23649=CARTESIAN_POINT('',(28.0133013427258,1.90995901823044,42.));
#23650=CARTESIAN_POINT('Origin',(29.667462259531,2.5,42.));
#23651=CARTESIAN_POINT('',(29.667462259531,2.5,41.7));
#23652=CARTESIAN_POINT('',(29.667462259531,2.5,42.));
#23653=CARTESIAN_POINT('',(29.667462259531,2.5,41.7));
#23654=CARTESIAN_POINT('Origin',(25.7042973488569,2.5,42.));
#23655=CARTESIAN_POINT('',(25.7042973488569,2.5,41.7));
#23656=CARTESIAN_POINT('',(25.7042973488569,2.5,42.));
#23657=CARTESIAN_POINT('',(25.7042973488569,2.5,41.7));
#23658=CARTESIAN_POINT('Origin',(25.7042973488569,1.90995901823044,42.));
#23659=CARTESIAN_POINT('',(25.7042973488569,1.90995901823044,41.7));
#23660=CARTESIAN_POINT('',(25.7042973488569,1.90995901823044,42.));
#23661=CARTESIAN_POINT('',(25.7042973488569,1.90995901823044,41.7));
#23662=CARTESIAN_POINT('Origin',(27.3516370356083,1.90995901823044,42.));
#23663=CARTESIAN_POINT('',(27.3516370356083,1.90995901823044,41.7));
#23664=CARTESIAN_POINT('',(27.3516370356083,1.90995901823044,42.));
#23665=CARTESIAN_POINT('',(27.3516370356083,1.90995901823044,41.7));
#23666=CARTESIAN_POINT('Origin',(27.3516370356083,-2.5,42.));
#23667=CARTESIAN_POINT('',(27.3516370356083,-2.5,41.7));
#23668=CARTESIAN_POINT('',(27.3516370356083,-2.5,42.));
#23669=CARTESIAN_POINT('',(27.3516370356083,-2.5,41.7));
#23670=CARTESIAN_POINT('Origin',(28.0133013427258,-2.5,42.));
#23671=CARTESIAN_POINT('',(28.0133013427258,-2.5,41.7));
#23672=CARTESIAN_POINT('',(28.0133013427258,-2.5,42.));
#23673=CARTESIAN_POINT('',(28.0133013427258,-2.5,41.7));
#23674=CARTESIAN_POINT('Origin',(28.0133013427258,1.90995901823044,42.));
#23675=CARTESIAN_POINT('',(28.0133013427258,1.90995901823044,41.7));
#23676=CARTESIAN_POINT('Origin',(27.685879804194,0.,41.7));
#23677=CARTESIAN_POINT('Ctrl Pts',(20.4519100487232,-2.14699864387512,42.));
#23678=CARTESIAN_POINT('Ctrl Pts',(20.4519100487232,-2.14699864387512,41.7));
#23679=CARTESIAN_POINT('Ctrl Pts',(19.9982947669923,-1.7087310552597,42.));
#23680=CARTESIAN_POINT('Ctrl Pts',(19.9982947669923,-1.7087310552597,41.7));
#23681=CARTESIAN_POINT('Ctrl Pts',(19.9982947669923,-1.05388820171356,42.));
#23682=CARTESIAN_POINT('Ctrl Pts',(19.9982947669923,-1.05388820171356,41.7));
#23683=CARTESIAN_POINT('',(20.4519100487232,-2.14699864387512,41.7));
#23684=CARTESIAN_POINT('',(20.4519100487232,-2.14699864387512,42.));
#23685=CARTESIAN_POINT('',(19.9982947669923,-1.05388820171356,41.7));
#23686=CARTESIAN_POINT('Ctrl Pts',(20.4519100487232,-2.14699864387512,41.7));
#23687=CARTESIAN_POINT('Ctrl Pts',(19.9982947669923,-1.7087310552597,41.7));
#23688=CARTESIAN_POINT('Ctrl Pts',(19.9982947669923,-1.05388820171356,41.7));
#23689=CARTESIAN_POINT('',(19.9982947669923,-1.05388820171356,42.));
#23690=CARTESIAN_POINT('Ctrl Pts',(21.6456344723701,-2.58526623249054,42.));
#23691=CARTESIAN_POINT('Ctrl Pts',(21.6456344723701,-2.58526623249054,41.7));
#23692=CARTESIAN_POINT('Ctrl Pts',(20.9055253863335,-2.58526623249054,42.));
#23693=CARTESIAN_POINT('Ctrl Pts',(20.9055253863335,-2.58526623249054,41.7));
#23694=CARTESIAN_POINT('Ctrl Pts',(20.4519100487232,-2.14699864387512,42.));
#23695=CARTESIAN_POINT('Ctrl Pts',(20.4519100487232,-2.14699864387512,41.7));
#23696=CARTESIAN_POINT('',(21.6456344723701,-2.58526623249054,41.7));
#23697=CARTESIAN_POINT('',(21.6456344723701,-2.58526623249054,42.));
#23698=CARTESIAN_POINT('Ctrl Pts',(21.6456344723701,-2.58526623249054,41.7));
#23699=CARTESIAN_POINT('Ctrl Pts',(20.9055253863335,-2.58526623249054,41.7));
#23700=CARTESIAN_POINT('Ctrl Pts',(20.4519100487232,-2.14699864387512,41.7));
#23701=CARTESIAN_POINT('Ctrl Pts',(22.8393588960171,-2.14870393276215,42.));
#23702=CARTESIAN_POINT('Ctrl Pts',(22.8393588960171,-2.14870393276215,41.7));
#23703=CARTESIAN_POINT('Ctrl Pts',(22.3857437074184,-2.58526623249054,42.));
#23704=CARTESIAN_POINT('Ctrl Pts',(22.3857437074184,-2.58526623249054,41.7));
#23705=CARTESIAN_POINT('Ctrl Pts',(21.6456344723701,-2.58526623249054,42.));
#23706=CARTESIAN_POINT('Ctrl Pts',(21.6456344723701,-2.58526623249054,41.7));
#23707=CARTESIAN_POINT('',(22.8393588960171,-2.14870393276215,41.7));
#23708=CARTESIAN_POINT('',(22.8393588960171,-2.14870393276215,42.));
#23709=CARTESIAN_POINT('Ctrl Pts',(22.8393588960171,-2.14870393276215,41.7));
#23710=CARTESIAN_POINT('Ctrl Pts',(22.3857437074184,-2.58526623249054,41.7));
#23711=CARTESIAN_POINT('Ctrl Pts',(21.6456344723701,-2.58526623249054,41.7));
#23712=CARTESIAN_POINT('Ctrl Pts',(23.2929743826389,-1.07094138860703,42.));
#23713=CARTESIAN_POINT('Ctrl Pts',(23.2929743826389,-1.07094138860703,41.7));
#23714=CARTESIAN_POINT('Ctrl Pts',(23.2929743826389,-1.71214163303375,42.));
#23715=CARTESIAN_POINT('Ctrl Pts',(23.2929743826389,-1.71214163303375,41.7));
#23716=CARTESIAN_POINT('Ctrl Pts',(22.8393588960171,-2.14870393276215,42.));
#23717=CARTESIAN_POINT('Ctrl Pts',(22.8393588960171,-2.14870393276215,41.7));
#23718=CARTESIAN_POINT('',(23.2929743826389,-1.07094138860703,41.7));
#23719=CARTESIAN_POINT('',(23.2929743826389,-1.07094138860703,42.));
#23720=CARTESIAN_POINT('Ctrl Pts',(23.2929743826389,-1.07094138860703,41.7));
#23721=CARTESIAN_POINT('Ctrl Pts',(23.2929743826389,-1.71214163303375,41.7));
#23722=CARTESIAN_POINT('Ctrl Pts',(22.8393588960171,-2.14870393276215,41.7));
#23723=CARTESIAN_POINT('Ctrl Pts',(23.0525241792202,-0.272851288318634,
42.));
#23724=CARTESIAN_POINT('Ctrl Pts',(23.0525241792202,-0.272851288318634,
41.7));
#23725=CARTESIAN_POINT('Ctrl Pts',(23.2929743826389,-0.607094168663025,
42.));
#23726=CARTESIAN_POINT('Ctrl Pts',(23.2929743826389,-0.607094168663025,
41.7));
#23727=CARTESIAN_POINT('Ctrl Pts',(23.2929743826389,-1.07094138860703,42.));
#23728=CARTESIAN_POINT('Ctrl Pts',(23.2929743826389,-1.07094138860703,41.7));
#23729=CARTESIAN_POINT('',(23.0525241792202,-0.272851288318634,41.7));
#23730=CARTESIAN_POINT('',(23.0525241792202,-0.272851288318634,42.));
#23731=CARTESIAN_POINT('Ctrl Pts',(23.0525241792202,-0.272851288318634,
41.7));
#23732=CARTESIAN_POINT('Ctrl Pts',(23.2929743826389,-0.607094168663025,
41.7));
#23733=CARTESIAN_POINT('Ctrl Pts',(23.2929743826389,-1.07094138860703,41.7));
#23734=CARTESIAN_POINT('Ctrl Pts',(22.3516373336315,0.211459994316101,42.));
#23735=CARTESIAN_POINT('Ctrl Pts',(22.3516373336315,0.211459994316101,41.7));
#23736=CARTESIAN_POINT('Ctrl Pts',(22.8120739758015,0.0613915920257568,
42.));
#23737=CARTESIAN_POINT('Ctrl Pts',(22.8120739758015,0.0613915920257568,
41.7));
#23738=CARTESIAN_POINT('Ctrl Pts',(23.0525241792202,-0.272851288318634,
42.));
#23739=CARTESIAN_POINT('Ctrl Pts',(23.0525241792202,-0.272851288318634,
41.7));
#23740=CARTESIAN_POINT('',(22.3516373336315,0.211459994316101,41.7));
#23741=CARTESIAN_POINT('',(22.3516373336315,0.211459994316101,42.));
#23742=CARTESIAN_POINT('Ctrl Pts',(22.3516373336315,0.211459994316101,41.7));
#23743=CARTESIAN_POINT('Ctrl Pts',(22.8120739758015,0.0613915920257568,
41.7));
#23744=CARTESIAN_POINT('Ctrl Pts',(23.0525241792202,-0.272851288318634,
41.7));
#23745=CARTESIAN_POINT('Ctrl Pts',(22.9058663547039,0.608799457550049,42.));
#23746=CARTESIAN_POINT('Ctrl Pts',(22.9058663547039,0.608799457550049,41.7));
#23747=CARTESIAN_POINT('Ctrl Pts',(22.7233971655369,0.351296067237854,42.));
#23748=CARTESIAN_POINT('Ctrl Pts',(22.7233971655369,0.351296067237854,41.7));
#23749=CARTESIAN_POINT('Ctrl Pts',(22.3516373336315,0.211459994316101,42.));
#23750=CARTESIAN_POINT('Ctrl Pts',(22.3516373336315,0.211459994316101,41.7));
#23751=CARTESIAN_POINT('',(22.9058663547039,0.608799457550049,41.7));
#23752=CARTESIAN_POINT('',(22.9058663547039,0.608799457550049,42.));
#23753=CARTESIAN_POINT('Ctrl Pts',(22.9058663547039,0.608799457550049,41.7));
#23754=CARTESIAN_POINT('Ctrl Pts',(22.7233971655369,0.351296067237854,41.7));
#23755=CARTESIAN_POINT('Ctrl Pts',(22.3516373336315,0.211459994316101,41.7));
#23756=CARTESIAN_POINT('Ctrl Pts',(23.0883358418941,1.21418833732605,42.));
#23757=CARTESIAN_POINT('Ctrl Pts',(23.0883358418941,1.21418833732605,41.7));
#23758=CARTESIAN_POINT('Ctrl Pts',(23.0883358418941,0.866302847862244,42.));
#23759=CARTESIAN_POINT('Ctrl Pts',(23.0883358418941,0.866302847862244,41.7));
#23760=CARTESIAN_POINT('Ctrl Pts',(22.9058663547039,0.608799457550049,42.));
#23761=CARTESIAN_POINT('Ctrl Pts',(22.9058663547039,0.608799457550049,41.7));
#23762=CARTESIAN_POINT('',(23.0883358418941,1.21418833732605,41.7));
#23763=CARTESIAN_POINT('',(23.0883358418941,1.21418833732605,42.));
#23764=CARTESIAN_POINT('Ctrl Pts',(23.0883358418941,1.21418833732605,41.7));
#23765=CARTESIAN_POINT('Ctrl Pts',(23.0883358418941,0.866302847862244,41.7));
#23766=CARTESIAN_POINT('Ctrl Pts',(22.9058663547039,0.608799457550049,41.7));
#23767=CARTESIAN_POINT('Ctrl Pts',(22.68929079175,2.14017748832703,42.));
#23768=CARTESIAN_POINT('Ctrl Pts',(22.68929079175,2.14017748832703,41.7));
#23769=CARTESIAN_POINT('Ctrl Pts',(23.0883358418941,1.75989091396332,42.));
#23770=CARTESIAN_POINT('Ctrl Pts',(23.0883358418941,1.75989091396332,41.7));
#23771=CARTESIAN_POINT('Ctrl Pts',(23.0883358418941,1.21418833732605,42.));
#23772=CARTESIAN_POINT('Ctrl Pts',(23.0883358418941,1.21418833732605,41.7));
#23773=CARTESIAN_POINT('',(22.68929079175,2.14017748832703,41.7));
#23774=CARTESIAN_POINT('',(22.68929079175,2.14017748832703,42.));
#23775=CARTESIAN_POINT('Ctrl Pts',(22.68929079175,2.14017748832703,41.7));
#23776=CARTESIAN_POINT('Ctrl Pts',(23.0883358418941,1.75989091396332,41.7));
#23777=CARTESIAN_POINT('Ctrl Pts',(23.0883358418941,1.21418833732605,41.7));
#23778=CARTESIAN_POINT('Ctrl Pts',(21.6354024410248,2.52046346664429,42.));
#23779=CARTESIAN_POINT('Ctrl Pts',(21.6354024410248,2.52046346664429,41.7));
#23780=CARTESIAN_POINT('Ctrl Pts',(22.2902457416058,2.52046346664429,42.));
#23781=CARTESIAN_POINT('Ctrl Pts',(22.2902457416058,2.52046346664429,41.7));
#23782=CARTESIAN_POINT('Ctrl Pts',(22.68929079175,2.14017748832703,42.));
#23783=CARTESIAN_POINT('Ctrl Pts',(22.68929079175,2.14017748832703,41.7));
#23784=CARTESIAN_POINT('',(21.6354024410248,2.52046346664429,41.7));
#23785=CARTESIAN_POINT('',(21.6354024410248,2.52046346664429,42.));
#23786=CARTESIAN_POINT('Ctrl Pts',(21.6354024410248,2.52046346664429,41.7));
#23787=CARTESIAN_POINT('Ctrl Pts',(22.2902457416058,2.52046346664429,41.7));
#23788=CARTESIAN_POINT('Ctrl Pts',(22.68929079175,2.14017748832703,41.7));
#23789=CARTESIAN_POINT('Ctrl Pts',(20.5917463451624,2.14870393276215,42.));
#23790=CARTESIAN_POINT('Ctrl Pts',(20.5917463451624,2.14870393276215,41.7));
#23791=CARTESIAN_POINT('Ctrl Pts',(20.9839700162411,2.52046346664429,42.));
#23792=CARTESIAN_POINT('Ctrl Pts',(20.9839700162411,2.52046346664429,41.7));
#23793=CARTESIAN_POINT('Ctrl Pts',(21.6354024410248,2.52046346664429,42.));
#23794=CARTESIAN_POINT('Ctrl Pts',(21.6354024410248,2.52046346664429,41.7));
#23795=CARTESIAN_POINT('',(20.5917463451624,2.14870393276215,41.7));
#23796=CARTESIAN_POINT('',(20.5917463451624,2.14870393276215,42.));
#23797=CARTESIAN_POINT('Ctrl Pts',(20.5917463451624,2.14870393276215,41.7));
#23798=CARTESIAN_POINT('Ctrl Pts',(20.9839700162411,2.52046346664429,41.7));
#23799=CARTESIAN_POINT('Ctrl Pts',(21.6354024410248,2.52046346664429,41.7));
#23800=CARTESIAN_POINT('Ctrl Pts',(20.1995225995779,1.23124152421951,42.));
#23801=CARTESIAN_POINT('Ctrl Pts',(20.1995225995779,1.23124152421951,41.7));
#23802=CARTESIAN_POINT('Ctrl Pts',(20.1995225995779,1.77694410085678,42.));
#23803=CARTESIAN_POINT('Ctrl Pts',(20.1995225995779,1.77694410085678,41.7));
#23804=CARTESIAN_POINT('Ctrl Pts',(20.5917463451624,2.14870393276215,42.));
#23805=CARTESIAN_POINT('Ctrl Pts',(20.5917463451624,2.14870393276215,41.7));
#23806=CARTESIAN_POINT('',(20.1995225995779,1.23124152421951,41.7));
#23807=CARTESIAN_POINT('',(20.1995225995779,1.23124152421951,42.));
#23808=CARTESIAN_POINT('Ctrl Pts',(20.1995225995779,1.23124152421951,41.7));
#23809=CARTESIAN_POINT('Ctrl Pts',(20.1995225995779,1.77694410085678,41.7));
#23810=CARTESIAN_POINT('Ctrl Pts',(20.5917463451624,2.14870393276215,41.7));
#23811=CARTESIAN_POINT('Ctrl Pts',(20.3836972266436,0.610504746437073,42.));
#23812=CARTESIAN_POINT('Ctrl Pts',(20.3836972266436,0.610504746437073,41.7));
#23813=CARTESIAN_POINT('Ctrl Pts',(20.1995225995779,0.869713723659515,42.));
#23814=CARTESIAN_POINT('Ctrl Pts',(20.1995225995779,0.869713723659515,41.7));
#23815=CARTESIAN_POINT('Ctrl Pts',(20.1995225995779,1.23124152421951,42.));
#23816=CARTESIAN_POINT('Ctrl Pts',(20.1995225995779,1.23124152421951,41.7));
#23817=CARTESIAN_POINT('',(20.3836972266436,0.610504746437073,41.7));
#23818=CARTESIAN_POINT('',(20.3836972266436,0.610504746437073,42.));
#23819=CARTESIAN_POINT('Ctrl Pts',(20.3836972266436,0.610504746437073,41.7));
#23820=CARTESIAN_POINT('Ctrl Pts',(20.1995225995779,0.869713723659515,41.7));
#23821=CARTESIAN_POINT('Ctrl Pts',(20.1995225995779,1.23124152421951,41.7));
#23822=CARTESIAN_POINT('Ctrl Pts',(20.94986371696,0.211459994316101,42.));
#23823=CARTESIAN_POINT('Ctrl Pts',(20.94986371696,0.211459994316101,41.7));
#23824=CARTESIAN_POINT('Ctrl Pts',(20.5678718537092,0.351296067237854,42.));
#23825=CARTESIAN_POINT('Ctrl Pts',(20.5678718537092,0.351296067237854,41.7));
#23826=CARTESIAN_POINT('Ctrl Pts',(20.3836972266436,0.610504746437073,42.));
#23827=CARTESIAN_POINT('Ctrl Pts',(20.3836972266436,0.610504746437073,41.7));
#23828=CARTESIAN_POINT('',(20.94986371696,0.211459994316101,41.7));
#23829=CARTESIAN_POINT('',(20.94986371696,0.211459994316101,42.));
#23830=CARTESIAN_POINT('Ctrl Pts',(20.94986371696,0.211459994316101,41.7));
#23831=CARTESIAN_POINT('Ctrl Pts',(20.5678718537092,0.351296067237854,41.7));
#23832=CARTESIAN_POINT('Ctrl Pts',(20.3836972266436,0.610504746437073,41.7));
#23833=CARTESIAN_POINT('Ctrl Pts',(20.2455662563443,-0.237039625644684,
42.));
#23834=CARTESIAN_POINT('Ctrl Pts',(20.2455662563443,-0.237039625644684,
41.7));
#23835=CARTESIAN_POINT('Ctrl Pts',(20.4928377270699,0.0920873880386353,
42.));
#23836=CARTESIAN_POINT('Ctrl Pts',(20.4928377270699,0.0920873880386353,
41.7));
#23837=CARTESIAN_POINT('Ctrl Pts',(20.94986371696,0.211459994316101,42.));
#23838=CARTESIAN_POINT('Ctrl Pts',(20.94986371696,0.211459994316101,41.7));
#23839=CARTESIAN_POINT('',(20.2455662563443,-0.237039625644684,41.7));
#23840=CARTESIAN_POINT('',(20.2455662563443,-0.237039625644684,42.));
#23841=CARTESIAN_POINT('Ctrl Pts',(20.2455662563443,-0.237039625644684,
41.7));
#23842=CARTESIAN_POINT('Ctrl Pts',(20.4928377270699,0.0920873880386353,
41.7));
#23843=CARTESIAN_POINT('Ctrl Pts',(20.94986371696,0.211459994316101,41.7));
#23844=CARTESIAN_POINT('Ctrl Pts',(19.9982947669923,-1.05388820171356,42.));
#23845=CARTESIAN_POINT('Ctrl Pts',(19.9982947669923,-1.05388820171356,41.7));
#23846=CARTESIAN_POINT('Ctrl Pts',(19.9982947669923,-0.566166639328003,
42.));
#23847=CARTESIAN_POINT('Ctrl Pts',(19.9982947669923,-0.566166639328003,
41.7));
#23848=CARTESIAN_POINT('Ctrl Pts',(20.2455662563443,-0.237039625644684,
42.));
#23849=CARTESIAN_POINT('Ctrl Pts',(20.2455662563443,-0.237039625644684,
41.7));
#23850=CARTESIAN_POINT('Ctrl Pts',(19.9982947669923,-1.05388820171356,41.7));
#23851=CARTESIAN_POINT('Ctrl Pts',(19.9982947669923,-0.566166639328003,
41.7));
#23852=CARTESIAN_POINT('Ctrl Pts',(20.2455662563443,-0.237039625644684,
41.7));
#23853=CARTESIAN_POINT('Origin',(21.6456345748156,-0.0324013829231262,41.7));
#23854=CARTESIAN_POINT('Origin',(39.0330834686756,-2.5,42.));
#23855=CARTESIAN_POINT('',(39.0330834686756,-2.5,41.7));
#23856=CARTESIAN_POINT('',(39.0330834686756,-2.5,42.));
#23857=CARTESIAN_POINT('',(36.4068896323442,1.42905861139297,41.7));
#23858=CARTESIAN_POINT('',(39.0330834686756,-2.5,41.7));
#23859=CARTESIAN_POINT('',(36.4068896323442,1.42905861139297,42.));
#23860=CARTESIAN_POINT('Origin',(39.7118009626865,-2.5,42.));
#23861=CARTESIAN_POINT('',(39.7118009626865,-2.5,41.7));
#23862=CARTESIAN_POINT('',(39.7118009626865,-2.5,42.));
#23863=CARTESIAN_POINT('',(39.7118009626865,-2.5,41.7));
#23864=CARTESIAN_POINT('Origin',(39.7118009626865,2.5,42.));
#23865=CARTESIAN_POINT('',(39.7118009626865,2.5,41.7));
#23866=CARTESIAN_POINT('',(39.7118009626865,2.5,42.));
#23867=CARTESIAN_POINT('',(39.7118009626865,2.5,41.7));
#23868=CARTESIAN_POINT('Origin',(39.0774215757847,2.5,42.));
#23869=CARTESIAN_POINT('',(39.0774215757847,2.5,41.7));
#23870=CARTESIAN_POINT('',(39.0774215757847,2.5,42.));
#23871=CARTESIAN_POINT('',(39.0774215757847,2.5,41.7));
#23872=CARTESIAN_POINT('Origin',(39.0774215757847,-1.42564833164215,42.));
#23873=CARTESIAN_POINT('',(39.0774215757847,-1.42564833164215,41.7));
#23874=CARTESIAN_POINT('',(39.0774215757847,-1.42564833164215,42.));
#23875=CARTESIAN_POINT('',(39.0774215757847,-1.42564833164215,41.7));
#23876=CARTESIAN_POINT('Origin',(36.4512279629707,2.5,42.));
#23877=CARTESIAN_POINT('',(36.4512279629707,2.5,41.7));
#23878=CARTESIAN_POINT('',(36.4512279629707,2.5,42.));
#23879=CARTESIAN_POINT('',(36.4512279629707,2.5,41.7));
#23880=CARTESIAN_POINT('Origin',(35.772510394454,2.5,42.));
#23881=CARTESIAN_POINT('',(35.772510394454,2.5,41.7));
#23882=CARTESIAN_POINT('',(35.772510394454,2.5,42.));
#23883=CARTESIAN_POINT('',(35.772510394454,2.5,41.7));
#23884=CARTESIAN_POINT('Origin',(35.772510394454,-2.5,42.));
#23885=CARTESIAN_POINT('',(35.772510394454,-2.5,41.7));
#23886=CARTESIAN_POINT('',(35.772510394454,-2.5,42.));
#23887=CARTESIAN_POINT('',(35.772510394454,-2.5,41.7));
#23888=CARTESIAN_POINT('Origin',(36.4068896323442,-2.5,42.));
#23889=CARTESIAN_POINT('',(36.4068896323442,-2.5,41.7));
#23890=CARTESIAN_POINT('',(36.4068896323442,-2.5,42.));
#23891=CARTESIAN_POINT('',(36.4068896323442,-2.5,41.7));
#23892=CARTESIAN_POINT('Origin',(36.4068896323442,1.42905861139297,42.));
#23893=CARTESIAN_POINT('',(36.4068896323442,1.42905861139297,41.7));
#23894=CARTESIAN_POINT('Origin',(37.7421556785703,0.,41.7));
#23895=CARTESIAN_POINT('Origin',(15.,0.,0.));
#23896=CARTESIAN_POINT('',(9.9,-3.73517273739943E-16,3.05));
#23897=CARTESIAN_POINT('',(15.,3.73517273739943E-16,3.05));
#23898=CARTESIAN_POINT('Origin',(9.9,0.,0.));
#23899=CARTESIAN_POINT('Origin',(9.9,0.,0.));
#23900=CARTESIAN_POINT('Origin',(91.6,0.,0.));
#23901=CARTESIAN_POINT('',(91.1,-21.05,-2.57788151220518E-15));
#23902=CARTESIAN_POINT('Origin',(91.1,0.,0.));
#23903=CARTESIAN_POINT('',(91.6,-21.525,-2.63605223516468E-15));
#23904=CARTESIAN_POINT('Origin',(80.05,0.,0.));
#23905=CARTESIAN_POINT('',(80.05,-21.05,-2.57788151220518E-15));
#23906=CARTESIAN_POINT('Origin',(42.,22.,8.5));
#23907=CARTESIAN_POINT('Origin',(84.,-22.,22.));
#23908=CARTESIAN_POINT('Origin',(42.,22.,8.5));
#45194=UNCERTAINTY_MEASURE_WITH_UNIT(LENGTH_MEASURE(0.01),#45237,
'DISTANCE_ACCURACY_VALUE',
'Maximum model space distance between geometric entities at asserted c
onnectivities');
#45214=UNCERTAINTY_MEASURE_WITH_UNIT(LENGTH_MEASURE(0.01),#45237,
'DISTANCE_ACCURACY_VALUE',
'Maximum model space distance between geometric entities at asserted c
onnectivities');
#45216=(
GEOMETRIC_REPRESENTATION_CONTEXT(3)
GLOBAL_UNCERTAINTY_ASSIGNED_CONTEXT((#45194))
GLOBAL_UNIT_ASSIGNED_CONTEXT((#45237,#45239,#45240))
REPRESENTATION_CONTEXT('','3D')
);
#45236=(
GEOMETRIC_REPRESENTATION_CONTEXT(3)
GLOBAL_UNCERTAINTY_ASSIGNED_CONTEXT((#45214))
GLOBAL_UNIT_ASSIGNED_CONTEXT((#45237,#45239,#45240))
REPRESENTATION_CONTEXT('','3D')
);
#45237=(
LENGTH_UNIT()
NAMED_UNIT(*)
SI_UNIT(.MILLI.,.METRE.)
);
#45239=(
NAMED_UNIT(*)
PLANE_ANGLE_UNIT()
SI_UNIT($,.RADIAN.)
);
#45240=(
NAMED_UNIT(*)
SI_UNIT($,.STERADIAN.)
SOLID_ANGLE_UNIT()
);
#45242=SHAPE_DEFINITION_REPRESENTATION(#45263,#45314);
#45263=PRODUCT_DEFINITION_SHAPE('',$,#45336);
#45314=SHAPE_REPRESENTATION('',(#16759),#45216);
#45334=PRODUCT_DEFINITION_CONTEXT('part definition',#45399,'design');
#45336=PRODUCT_DEFINITION('2026-10-25-23-38-11-368',
'01_Pincer_Head_C-Frame',#45357,#45334);
#45357=PRODUCT_DEFINITION_FORMATION('',$,#45402);
#45399=APPLICATION_CONTEXT(
'Core Data for Automotive Mechanical Design Process');
#45400=PRODUCT_CONTEXT('part definition',#45399,'mechanical');
#45402=PRODUCT('2026-10-25-23-38-11-368','01_Pincer_Head_C-Frame',$,(#45400));
#45457=COLOUR_RGB('Dark Blue',0.08,0.2,0.34);
#45458=FILL_AREA_STYLE_COLOUR('',#45457);
#45459=FILL_AREA_STYLE('',(#45458));
#45460=SURFACE_STYLE_FILL_AREA(#45459);
#45461=SURFACE_SIDE_STYLE('',(#45460));
#45462=SURFACE_STYLE_USAGE(.BOTH.,#45461);
#45463=PRESENTATION_STYLE_ASSIGNMENT((#45462));
ENDSEC;
END-ISO-10303-21;
